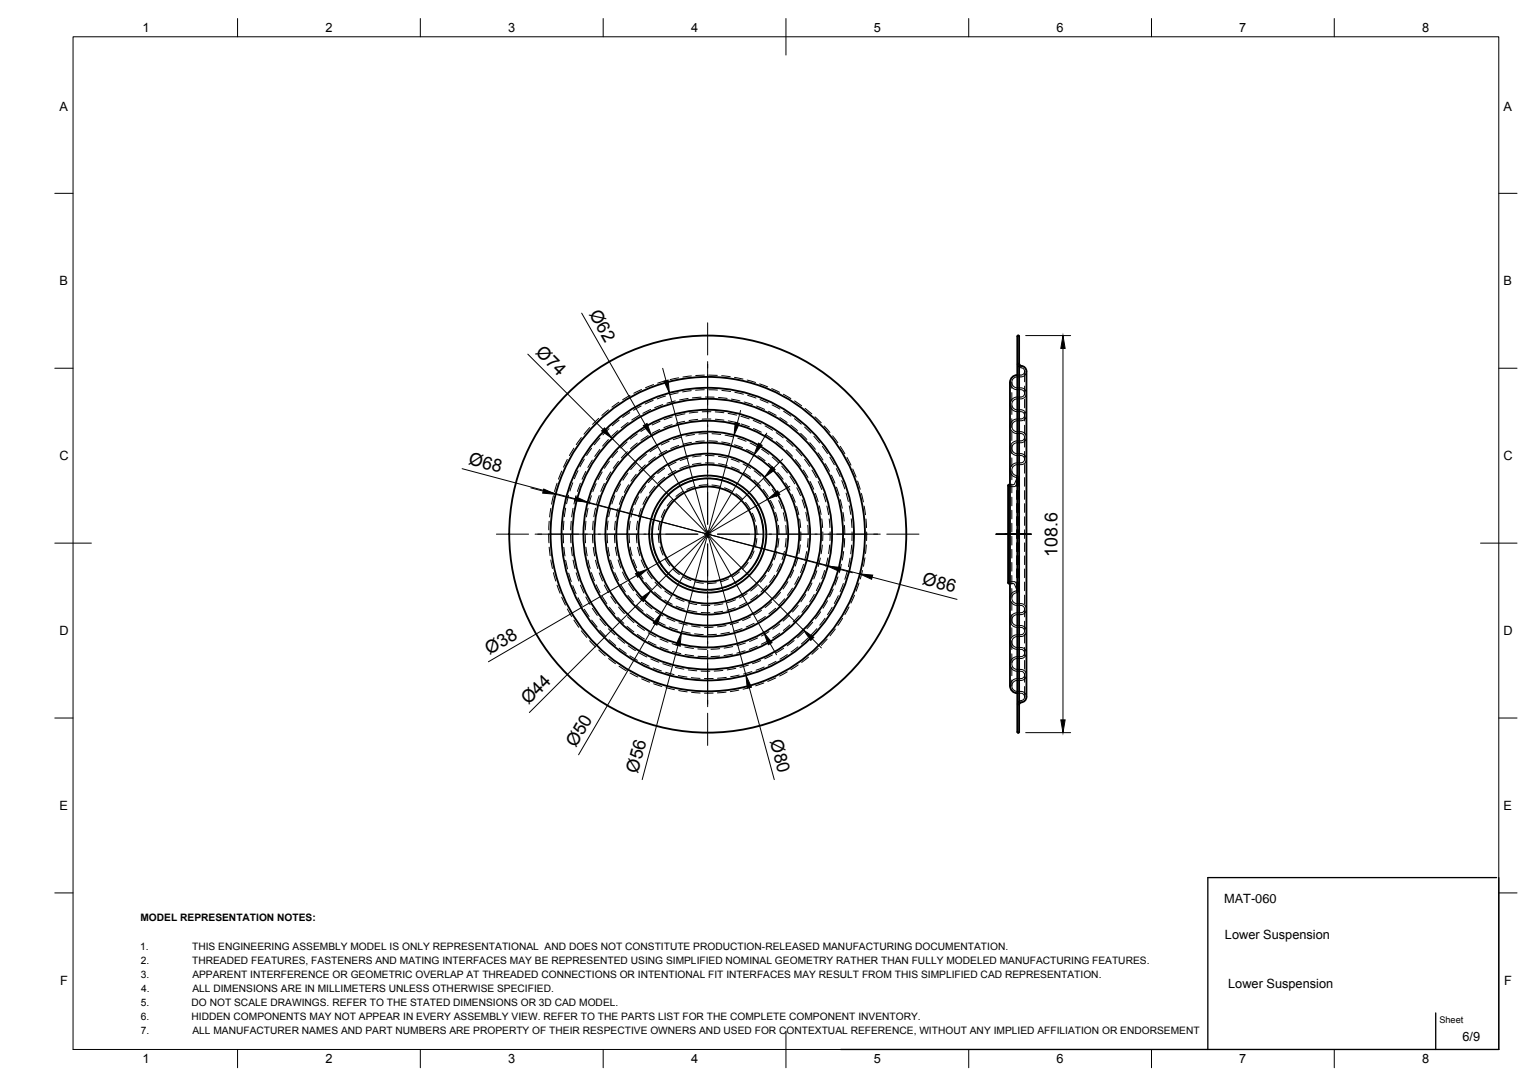
ISO-10303-21;
HEADER;
FILE_DESCRIPTION (('STEP AP214'),
    '1' );
FILE_NAME ('Lower Suspension.step',
    '2026-10-29T23:46:56',
    ( '' ),
    ( '' ),
    'SwSTEP 2.0',
    'SolidWorks 2020',
    '' );
FILE_SCHEMA (( 'AUTOMOTIVE_DESIGN' ));
ENDSEC;

DATA;
#3=CARTESIAN_POINT ( 'NONE',  ( -8.402144023942796025, 14.86454579224779948, 47.04930799450052348 ) ) ;
#7=DIRECTION ( 'NONE',  ( -0.000000000000000000, -1.000000000000000000, 0.000000000000000000 ) ) ;
#16=CIRCLE ( 'NONE', #21997, 37.50000000000000711 ) ;
#18=EDGE_CURVE ( 'NONE', #23289, #31921, #28501, .T. ) ;
#33=EDGE_CURVE ( 'NONE', #28622, #18652, #13708, .T. ) ;
#61=DIRECTION ( 'NONE',  ( -0.000000000000000000, -1.000000000000000000, 0.000000000000000000 ) ) ;
#105=CYLINDRICAL_SURFACE ( 'NONE', #15721, 33.50000000000000000 ) ;
#126=EDGE_CURVE ( 'NONE', #12313, #19851, #23434, .T. ) ;
#127=FACE_OUTER_BOUND ( 'NONE', #2532, .T. ) ;
#144=AXIS2_PLACEMENT_3D ( 'NONE', #10705, #31040, #25937 ) ;
#148=DIRECTION ( 'NONE',  ( -1.000000000000000000, 0.000000000000000000, 0.000000000000000000 ) ) ;
#159=CARTESIAN_POINT ( 'NONE',  ( 21.09785597605720753, 14.86454579224779948, 47.04930799450052348 ) ) ;
#160=CARTESIAN_POINT ( 'NONE',  ( 75.19785597605721250, 14.66454579224780019, 47.04930799450051637 ) ) ;
#161=EDGE_CURVE ( 'NONE', #17230, #26186, #19107, .T. ) ;
#163=VERTEX_POINT ( 'NONE', #26839 ) ;
#164=ORIENTED_EDGE ( 'NONE', *, *, #2840, .T. ) ;
#166=FACE_OUTER_BOUND ( 'NONE', #10063, .T. ) ;
#169=ORIENTED_EDGE ( 'NONE', *, *, #20266, .F. ) ;
#198=CIRCLE ( 'NONE', #29008, 34.00000000000000000 ) ;
#201=EDGE_CURVE ( 'NONE', #31745, #29739, #32095, .T. ) ;
#212=CARTESIAN_POINT ( 'NONE',  ( 21.09785597605720753, 15.23835801850285776, 47.04930799450052348 ) ) ;
#227=FACE_OUTER_BOUND ( 'NONE', #31629, .T. ) ;
#233=DIRECTION ( 'NONE',  ( -1.000000000000000000, 0.000000000000000000, 0.000000000000000000 ) ) ;
#234=AXIS2_PLACEMENT_3D ( 'NONE', #13203, #26134, #3648 ) ;
#238=ORIENTED_EDGE ( 'NONE', *, *, #2347, .F. ) ;
#241=AXIS2_PLACEMENT_3D ( 'NONE', #30077, #17255, #27274 ) ;
#242=AXIS2_PLACEMENT_3D ( 'NONE', #2741, #20287, #4883 ) ;
#243=DIRECTION ( 'NONE',  ( 0.000000000000000000, 0.000000000000000000, 1.000000000000000000 ) ) ;
#247=CARTESIAN_POINT ( 'NONE',  ( 42.59785597605719687, 13.86454579224779948, 47.04930799450052348 ) ) ;
#275=CARTESIAN_POINT ( 'NONE',  ( 64.59785597605720397, 13.86454579224779948, 47.04930799450051637 ) ) ;
#285=DIRECTION ( 'NONE',  ( -0.000000000000000000, -1.000000000000000000, 0.000000000000000000 ) ) ;
#294=VERTEX_POINT ( 'NONE', #26940 ) ;
#297=ORIENTED_EDGE ( 'NONE', *, *, #25455, .T. ) ;
#315=DIRECTION ( 'NONE',  ( -0.000000000000000000, -1.000000000000000000, 0.000000000000000000 ) ) ;
#319=DIRECTION ( 'NONE',  ( -1.224646799147353207E-16, 0.000000000000000000, -1.000000000000000000 ) ) ;
#332=DIRECTION ( 'NONE',  ( -0.000000000000000000, -1.000000000000000000, 0.000000000000000000 ) ) ;
#339=DIRECTION ( 'NONE',  ( -1.000000000000000000, 0.000000000000000000, 0.000000000000000000 ) ) ;
#344=DIRECTION ( 'NONE',  ( -0.000000000000000000, -1.000000000000000000, 0.000000000000000000 ) ) ;
#345=AXIS2_PLACEMENT_3D ( 'NONE', #21627, #16382, #28696 ) ;
#354=SURFACE_STYLE_FILL_AREA ( #4142 ) ;
#364=DIRECTION ( 'NONE',  ( -1.000000000000000000, 0.000000000000000000, 0.000000000000000000 ) ) ;
#374=CARTESIAN_POINT ( 'NONE',  ( -25.43703420551703687, 14.86454579224779948, 47.04930799450052348 ) ) ;
#380=CARTESIAN_POINT ( 'NONE',  ( -33.00214402394279745, 14.56454579224780055, 47.04930799450052348 ) ) ;
#385=DIRECTION ( 'NONE',  ( -0.000000000000000000, -1.000000000000000000, 0.000000000000000000 ) ) ;
#393=DIRECTION ( 'NONE',  ( -0.000000000000000000, -1.000000000000000000, 0.000000000000000000 ) ) ;
#399=ORIENTED_EDGE ( 'NONE', *, *, #19336, .T. ) ;
#402=VECTOR ( 'NONE', #29431, 1000.000000000000000 ) ;
#416=ADVANCED_FACE ( 'NONE', ( #13916 ), #14557, .T. ) ;
#419=CIRCLE ( 'NONE', #21369, 34.00000000000000000 ) ;
#431=ORIENTED_EDGE ( 'NONE', *, *, #27668, .F. ) ;
#455=CIRCLE ( 'NONE', #23507, 1.290569415042103207 ) ;
#463=CIRCLE ( 'NONE', #20375, 0.3999999999999975797 ) ;
#470=EDGE_LOOP ( 'NONE', ( #9443, #11981, #20479, #1663 ) ) ;
#490=VERTEX_POINT ( 'NONE', #19471 ) ;
#492=AXIS2_PLACEMENT_3D ( 'NONE', #30621, #8133, #15667 ) ;
#500=EDGE_LOOP ( 'NONE', ( #31319, #977, #18838, #21612 ) ) ;
#524=FACE_OUTER_BOUND ( 'NONE', #6231, .T. ) ;
#547=AXIS2_PLACEMENT_3D ( 'NONE', #22754, #7337, #22261 ) ;
#548=VECTOR ( 'NONE', #4777, 1000.000000000000000 ) ;
#572=DIRECTION ( 'NONE',  ( -0.000000000000000000, -1.000000000000000000, 0.000000000000000000 ) ) ;
#581=AXIS2_PLACEMENT_3D ( 'NONE', #5824, #5343, #30613 ) ;
#616=ADVANCED_FACE ( 'NONE', ( #14724 ), #105, .F. ) ;
#617=DIRECTION ( 'NONE',  ( -1.000000000000000000, 0.000000000000000000, 0.000000000000000000 ) ) ;
#620=EDGE_LOOP ( 'NONE', ( #3859, #30417, #14895, #17526 ) ) ;
#627=ORIENTED_EDGE ( 'NONE', *, *, #27698, .T. ) ;
#629=TOROIDAL_SURFACE ( 'NONE', #20027, 35.50000000000000711, 2.000000000000001776 ) ;
#634=DIRECTION ( 'NONE',  ( 0.000000000000000000, 0.000000000000000000, 1.000000000000000000 ) ) ;
#646=VECTOR ( 'NONE', #22286, 1000.000000000000000 ) ;
#659=ORIENTED_EDGE ( 'NONE', *, *, #25819, .T. ) ;
#663=VERTEX_POINT ( 'NONE', #19058 ) ;
#665=VERTEX_POINT ( 'NONE', #23832 ) ;
#676=DIRECTION ( 'NONE',  ( -1.000000000000000000, 0.000000000000000000, 0.000000000000000000 ) ) ;
#678=DIRECTION ( 'NONE',  ( -0.000000000000000000, -1.000000000000000000, 0.000000000000000000 ) ) ;
#692=VECTOR ( 'NONE', #11554, 1000.000000000000000 ) ;
#706=CARTESIAN_POINT ( 'NONE',  ( 21.09785597605720753, 14.86454579224779948, 47.04930799450052348 ) ) ;
#710=EDGE_CURVE ( 'NONE', #26545, #16815, #18901, .T. ) ;
#733=CARTESIAN_POINT ( 'NONE',  ( -4.402144023942796025, 14.86454579224779948, 47.04930799450052348 ) ) ;
#742=DIRECTION ( 'NONE',  ( -1.000000000000000000, 0.000000000000000000, 0.000000000000000000 ) ) ;
#745=ORIENTED_EDGE ( 'NONE', *, *, #29770, .T. ) ;
#764=EDGE_LOOP ( 'NONE', ( #11253, #25732, #6784, #15942 ) ) ;
#772=DIRECTION ( 'NONE',  ( -1.224646799147353207E-16, 0.000000000000000000, -1.000000000000000000 ) ) ;
#775=DIRECTION ( 'NONE',  ( -0.000000000000000000, -1.000000000000000000, 0.000000000000000000 ) ) ;
#783=AXIS2_PLACEMENT_3D ( 'NONE', #18069, #31044, #28097 ) ;
#795=TOROIDAL_SURFACE ( 'NONE', #23343, 14.00178401536290806, 0.5000000000000004441 ) ;
#801=AXIS2_PLACEMENT_3D ( 'NONE', #9771, #4184, #12401 ) ;
#817=DIRECTION ( 'NONE',  ( -0.000000000000000000, -1.000000000000000000, 0.000000000000000000 ) ) ;
#826=ORIENTED_EDGE ( 'NONE', *, *, #5317, .F. ) ;
#829=DIRECTION ( 'NONE',  ( -1.224646799147353207E-16, 0.000000000000000000, -1.000000000000000000 ) ) ;
#847=CARTESIAN_POINT ( 'NONE',  ( 61.09785597605719687, 13.86454579224779948, 47.04930799450051637 ) ) ;
#861=EDGE_LOOP ( 'NONE', ( #24263, #7176, #5578, #9165 ) ) ;
#878=CARTESIAN_POINT ( 'NONE',  ( 67.13598395589038148, 13.95840365082257151, 47.04930799450051637 ) ) ;
#890=EDGE_CURVE ( 'NONE', #8606, #20520, #3192, .T. ) ;
#896=ORIENTED_EDGE ( 'NONE', *, *, #11025, .F. ) ;
#904=TOROIDAL_SURFACE ( 'NONE', #1959, 20.49999999999999645, 0.9999999999999974465 ) ;
#927=DIRECTION ( 'NONE',  ( 0.000000000000000000, 0.000000000000000000, 1.000000000000000000 ) ) ;
#953=EDGE_LOOP ( 'NONE', ( #21634, #23029, #10824, #21413 ) ) ;
#956=CIRCLE ( 'NONE', #32436, 40.00000000000000711 ) ;
#977=ORIENTED_EDGE ( 'NONE', *, *, #26692, .T. ) ;
#985=DIRECTION ( 'NONE',  ( -1.000000000000000000, 0.000000000000000000, 0.000000000000000000 ) ) ;
#996=ORIENTED_EDGE ( 'NONE', *, *, #8934, .T. ) ;
#1013=VERTEX_POINT ( 'NONE', #8550 ) ;
#1023=DIRECTION ( 'NONE',  ( -0.000000000000000000, -1.000000000000000000, 0.000000000000000000 ) ) ;
#1025=AXIS2_PLACEMENT_3D ( 'NONE', #1697, #21378, #8608 ) ;
#1049=CARTESIAN_POINT ( 'NONE',  ( 21.09785597605720753, 13.86454579224779948, 47.04930799450052348 ) ) ;
#1051=DIRECTION ( 'NONE',  ( -0.000000000000000000, -1.000000000000000000, 0.000000000000000000 ) ) ;
#1052=ORIENTED_EDGE ( 'NONE', *, *, #17154, .F. ) ;
#1079=CARTESIAN_POINT ( 'NONE',  ( 49.09785597605720397, 13.86454579224779948, 47.04930799450052348 ) ) ;
#1095=AXIS2_PLACEMENT_3D ( 'NONE', #18592, #20746, #15506 ) ;
#1102=ORIENTED_EDGE ( 'NONE', *, *, #890, .T. ) ;
#1120=CIRCLE ( 'NONE', #24168, 15.28675991284684343 ) ;
#1158=VERTEX_POINT ( 'NONE', #19679 ) ;
#1159=DIRECTION ( 'NONE',  ( -0.000000000000000000, -1.000000000000000000, 0.000000000000000000 ) ) ;
#1160=AXIS2_PLACEMENT_3D ( 'NONE', #19272, #11903, #31929 ) ;
#1191=EDGE_LOOP ( 'NONE', ( #20839, #14385, #18300, #16135 ) ) ;
#1192=CARTESIAN_POINT ( 'NONE',  ( 60.59785597605720397, 14.86454579224779948, 47.04930799450051637 ) ) ;
#1196=MANIFOLD_SOLID_BREP ( 'Stock-MAT-060-1', #11089 ) ;
#1206=LINE ( 'NONE', #30777, #8886 ) ;
#1212=ORIENTED_EDGE ( 'NONE', *, *, #28402, .T. ) ;
#1218=CONICAL_SURFACE ( 'NONE', #30581, 13.20165371409683708, 1.570144820418440945 ) ;
#1225=CIRCLE ( 'NONE', #32177, 46.53489018157424084 ) ;
#1227=FACE_OUTER_BOUND ( 'NONE', #10320, .T. ) ;
#1231=CARTESIAN_POINT ( 'NONE',  ( 61.09785597605721108, -5.098646251524523443, 47.04930799450051637 ) ) ;
#1242=ORIENTED_EDGE ( 'NONE', *, *, #28098, .T. ) ;
#1245=EDGE_CURVE ( 'NONE', #18233, #24509, #5247, .T. ) ;
#1256=ORIENTED_EDGE ( 'NONE', *, *, #4300, .T. ) ;
#1275=CIRCLE ( 'NONE', #11247, 46.03812797983318461 ) ;
#1281=CARTESIAN_POINT ( 'NONE',  ( 21.09785597605720753, 14.86454579224779948, 47.04930799450052348 ) ) ;
#1296=EDGE_CURVE ( 'NONE', #19168, #20299, #21078, .T. ) ;
#1321=DIRECTION ( 'NONE',  ( -0.000000000000000000, -1.000000000000000000, 0.000000000000000000 ) ) ;
#1332=AXIS2_PLACEMENT_3D ( 'NONE', #5299, #12197, #17433 ) ;
#1354=DIRECTION ( 'NONE',  ( 0.000000000000000000, 0.000000000000000000, 1.000000000000000000 ) ) ;
#1363=CARTESIAN_POINT ( 'NONE',  ( 21.09785597605720753, 15.11603238453479037, 47.04930799450052348 ) ) ;
#1377=CIRCLE ( 'NONE', #13975, 33.50000000000000000 ) ;
#1380=CIRCLE ( 'NONE', #19729, 54.10000000000000142 ) ;
#1387=DIRECTION ( 'NONE',  ( -1.000000000000000000, 0.000000000000000000, 0.000000000000000000 ) ) ;
#1388=ORIENTED_EDGE ( 'NONE', *, *, #25283, .F. ) ;
#1403=CARTESIAN_POINT ( 'NONE',  ( 59.59785597605720397, 13.86454579224779948, 47.04930799450051637 ) ) ;
#1415=ORIENTED_EDGE ( 'NONE', *, *, #9403, .T. ) ;
#1417=EDGE_LOOP ( 'NONE', ( #27072, #20083, #10401, #7399 ) ) ;
#1419=AXIS2_PLACEMENT_3D ( 'NONE', #21368, #5980, #13693 ) ;
#1426=CYLINDRICAL_SURFACE ( 'NONE', #18100, 34.00000000000000000 ) ;
#1432=ADVANCED_FACE ( 'NONE', ( #21127 ), #14282, .T. ) ;
#1433=ORIENTED_EDGE ( 'NONE', *, *, #18374, .T. ) ;
#1434=CARTESIAN_POINT ( 'NONE',  ( -33.20214402394279318, 14.66454579224779842, 47.04930799450052348 ) ) ;
#1437=CARTESIAN_POINT ( 'NONE',  ( 21.09785597605720753, 14.86454579224779948, 47.04930799450052348 ) ) ;
#1482=DIRECTION ( 'NONE',  ( -1.000000000000000000, 0.000000000000000000, 0.000000000000000000 ) ) ;
#1483=FACE_OUTER_BOUND ( 'NONE', #28820, .T. ) ;
#1488=CARTESIAN_POINT ( 'NONE',  ( 67.79048676704638865, 13.68462854903246573, 47.04930799450051637 ) ) ;
#1505=CARTESIAN_POINT ( 'NONE',  ( 7.596071960694297687, -5.098646251524523443, 47.04930799450052348 ) ) ;
#1514=CYLINDRICAL_SURFACE ( 'NONE', #21014, 54.30000000000000426 ) ;
#1522=CARTESIAN_POINT ( 'NONE',  ( 5.811096063210362317, 14.98269195386757602, 47.04930799450052348 ) ) ;
#1532=ORIENTED_EDGE ( 'NONE', *, *, #7122, .T. ) ;
#1537=ORIENTED_EDGE ( 'NONE', *, *, #16167, .F. ) ;
#1543=CYLINDRICAL_SURFACE ( 'NONE', #29774, 31.50000000000000000 ) ;
#1560=DIRECTION ( 'NONE',  ( -1.000000000000000000, 0.000000000000000000, 0.000000000000000000 ) ) ;
#1566=DIRECTION ( 'NONE',  ( -0.000000000000000000, -1.000000000000000000, 0.000000000000000000 ) ) ;
#1569=TOROIDAL_SURFACE ( 'NONE', #2111, 41.50000000000000000, 1.999999999999998224 ) ;
#1573=AXIS2_PLACEMENT_3D ( 'NONE', #2497, #15138, #12523 ) ;
#1585=AXIS2_PLACEMENT_3D ( 'NONE', #20292, #30323, #1560 ) ;
#1589=CYLINDRICAL_SURFACE ( 'NONE', #7623, 25.50000000000000355 ) ;
#1595=ORIENTED_EDGE ( 'NONE', *, *, #19844, .T. ) ;
#1613=DIRECTION ( 'NONE',  ( -0.000000000000000000, -1.000000000000000000, 0.000000000000000000 ) ) ;
#1616=DIRECTION ( 'NONE',  ( -0.000000000000000000, -1.000000000000000000, 0.000000000000000000 ) ) ;
#1618=ORIENTED_EDGE ( 'NONE', *, *, #5754, .T. ) ;
#1650=CYLINDRICAL_SURFACE ( 'NONE', #30215, 13.50178401536290806 ) ;
#1659=FACE_OUTER_BOUND ( 'NONE', #30379, .T. ) ;
#1663=ORIENTED_EDGE ( 'NONE', *, *, #18980, .T. ) ;
#1664=AXIS2_PLACEMENT_3D ( 'NONE', #2940, #17556, #20664 ) ;
#1692=CARTESIAN_POINT ( 'NONE',  ( 21.09785597605720753, 13.86454579224779948, 47.04930799450052348 ) ) ;
#1697=CARTESIAN_POINT ( 'NONE',  ( 21.09785597605720753, 14.86454579224779948, 47.04930799450052348 ) ) ;
#1705=EDGE_CURVE ( 'NONE', #3673, #7331, #3796, .T. ) ;
#1709=EDGE_CURVE ( 'NONE', #3673, #31872, #30548, .T. ) ;
#1719=CARTESIAN_POINT ( 'NONE',  ( 21.09785597605720753, 14.81645899701909563, 47.04930799450052348 ) ) ;
#1762=ORIENTED_EDGE ( 'NONE', *, *, #31648, .F. ) ;
#1768=DIRECTION ( 'NONE',  ( -0.000000000000000000, -1.000000000000000000, 0.000000000000000000 ) ) ;
#1776=CARTESIAN_POINT ( 'NONE',  ( -4.402144023942796025, 13.86454579224779948, 47.04930799450052348 ) ) ;
#1796=VERTEX_POINT ( 'NONE', #23083 ) ;
#1815=EDGE_CURVE ( 'NONE', #27059, #10602, #6898, .T. ) ;
#1835=ORIENTED_EDGE ( 'NONE', *, *, #9572, .T. ) ;
#1845=AXIS2_PLACEMENT_3D ( 'NONE', #30690, #5572, #3263 ) ;
#1856=ORIENTED_EDGE ( 'NONE', *, *, #8300, .T. ) ;
#1867=DIRECTION ( 'NONE',  ( 0.000000000000000000, 0.000000000000000000, 1.000000000000000000 ) ) ;
#1868=ORIENTED_EDGE ( 'NONE', *, *, #12433, .F. ) ;
#1875=DIRECTION ( 'NONE',  ( -1.224646799147353207E-16, 0.000000000000000000, -1.000000000000000000 ) ) ;
#1891=EDGE_CURVE ( 'NONE', #26545, #19851, #18412, .T. ) ;
#1902=ORIENTED_EDGE ( 'NONE', *, *, #24442, .T. ) ;
#1933=ORIENTED_EDGE ( 'NONE', *, *, #22375, .F. ) ;
#1935=DIRECTION ( 'NONE',  ( 0.9275012328650846793, -0.3738200944756017163, -1.135861416033449914E-16 ) ) ;
#1959=AXIS2_PLACEMENT_3D ( 'NONE', #7931, #27946, #15149 ) ;
#1971=ORIENTED_EDGE ( 'NONE', *, *, #4751, .T. ) ;
#2003=DIRECTION ( 'NONE',  ( -0.000000000000000000, -1.000000000000000000, 0.000000000000000000 ) ) ;
#2009=AXIS2_PLACEMENT_3D ( 'NONE', #9915, #29946, #12718 ) ;
#2010=AXIS2_PLACEMENT_3D ( 'NONE', #11975, #7046, #4265 ) ;
#2012=DIRECTION ( 'NONE',  ( -0.000000000000000000, -1.000000000000000000, 0.000000000000000000 ) ) ;
#2037=AXIS2_PLACEMENT_3D ( 'NONE', #3, #2629, #15747 ) ;
#2045=CARTESIAN_POINT ( 'NONE',  ( 34.09963999142011204, 15.70210863493540288, 47.04930799450052348 ) ) ;
#2053=CARTESIAN_POINT ( 'NONE',  ( 21.09785597605720753, 14.86454579224779948, 47.04930799450052348 ) ) ;
#2055=DIRECTION ( 'NONE',  ( -0.000000000000000000, -1.000000000000000000, 0.000000000000000000 ) ) ;
#2057=DIRECTION ( 'NONE',  ( -1.000000000000000000, 0.000000000000000000, 0.000000000000000000 ) ) ;
#2061=CIRCLE ( 'NONE', #20397, 27.49999999999999645 ) ;
#2071=ADVANCED_FACE ( 'NONE', ( #24704 ), #30126, .T. ) ;
#2079=DIRECTION ( 'NONE',  ( -1.000000000000000000, 0.000000000000000000, 0.000000000000000000 ) ) ;
#2088=DIRECTION ( 'NONE',  ( -1.224646799147353207E-16, 0.000000000000000000, -1.000000000000000000 ) ) ;
#2111=AXIS2_PLACEMENT_3D ( 'NONE', #4236, #18822, #16688 ) ;
#2112=TOROIDAL_SURFACE ( 'NONE', #7373, 13.30178401536290878, 0.2000000000000002609 ) ;
#2129=ORIENTED_EDGE ( 'NONE', *, *, #16040, .F. ) ;
#2142=CARTESIAN_POINT ( 'NONE',  ( 21.09785597605720753, 17.16467605102632632, 47.04930799450052348 ) ) ;
#2144=AXIS2_PLACEMENT_3D ( 'NONE', #28347, #8003, #23255 ) ;
#2159=EDGE_LOOP ( 'NONE', ( #14206, #9203, #31203, #26392 ) ) ;
#2173=DIRECTION ( 'NONE',  ( 0.000000000000000000, 0.000000000000000000, 1.000000000000000000 ) ) ;
#2182=ADVANCED_FACE ( 'NONE', ( #18269 ), #2727, .T. ) ;
#2186=DIRECTION ( 'NONE',  ( -0.000000000000000000, -1.000000000000000000, 0.000000000000000000 ) ) ;
#2193=ADVANCED_FACE ( 'NONE', ( #8276 ), #25512, .F. ) ;
#2199=CIRCLE ( 'NONE', #20531, 1.999999999999998224 ) ;
#2206=DIRECTION ( 'NONE',  ( -0.000000000000000000, -1.000000000000000000, 0.000000000000000000 ) ) ;
#2208=VECTOR ( 'NONE', #12644, 1000.000000000000000 ) ;
#2217=ORIENTED_EDGE ( 'NONE', *, *, #17290, .F. ) ;
#2219=CARTESIAN_POINT ( 'NONE',  ( 21.09785597605720753, -5.098646251524523443, 47.04930799450052348 ) ) ;
#2228=EDGE_CURVE ( 'NONE', #27481, #12804, #5802, .T. ) ;
#2242=CARTESIAN_POINT ( 'NONE',  ( 21.09785597605720753, -5.098646251524523443, 47.04930799450052348 ) ) ;
#2263=AXIS2_PLACEMENT_3D ( 'NONE', #4002, #14021, #19083 ) ;
#2272=CARTESIAN_POINT ( 'NONE',  ( 58.09785597605721108, -5.098646251524523443, 47.04930799450051637 ) ) ;
#2278=VECTOR ( 'NONE', #21411, 1000.000000000000000 ) ;
#2279=AXIS2_PLACEMENT_3D ( 'NONE', #14814, #20364, #10056 ) ;
#2288=LINE ( 'NONE', #30033, #23866 ) ;
#2307=TOROIDAL_SURFACE ( 'NONE', #26411, 15.35463912851480828, 0.6621856154243856984 ) ;
#2309=FACE_OUTER_BOUND ( 'NONE', #10411, .T. ) ;
#2311=EDGE_CURVE ( 'NONE', #7331, #3673, #14263, .T. ) ;
#2312=VERTEX_POINT ( 'NONE', #20333 ) ;
#2316=LINE ( 'NONE', #32192, #548 ) ;
#2328=ORIENTED_EDGE ( 'NONE', *, *, #25601, .T. ) ;
#2345=ADVANCED_FACE ( 'NONE', ( #27573 ), #1218, .F. ) ;
#2347=EDGE_CURVE ( 'NONE', #16477, #663, #28484, .T. ) ;
#2348=AXIS2_PLACEMENT_3D ( 'NONE', #11822, #13796, #19020 ) ;
#2350=EDGE_LOOP ( 'NONE', ( #17700, #31035, #31048, #18559 ) ) ;
#2353=DIRECTION ( 'NONE',  ( -1.000000000000000000, 0.000000000000000000, 0.000000000000000000 ) ) ;
#2357=AXIS2_PLACEMENT_3D ( 'NONE', #14559, #12104, #2413 ) ;
#2390=FACE_OUTER_BOUND ( 'NONE', #24514, .T. ) ;
#2393=DIRECTION ( 'NONE',  ( 1.000000000000000000, 0.000000000000000000, 0.000000000000000000 ) ) ;
#2407=ADVANCED_FACE ( 'NONE', ( #31327 ), #27966, .T. ) ;
#2413=DIRECTION ( 'NONE',  ( -1.000000000000000000, 0.000000000000000000, 0.000000000000000000 ) ) ;
#2439=EDGE_LOOP ( 'NONE', ( #4209, #25565, #3242, #13634 ) ) ;
#2441=VERTEX_POINT ( 'NONE', #13301 ) ;
#2443=AXIS2_PLACEMENT_3D ( 'NONE', #21790, #26722, #9166 ) ;
#2450=AXIS2_PLACEMENT_3D ( 'NONE', #27101, #16920, #14639 ) ;
#2463=DIRECTION ( 'NONE',  ( -0.000000000000000000, -1.000000000000000000, 0.000000000000000000 ) ) ;
#2468=CARTESIAN_POINT ( 'NONE',  ( -23.40214402394279247, 13.86454579224779948, 47.04930799450052348 ) ) ;
#2480=CARTESIAN_POINT ( 'NONE',  ( 21.09785597605720753, 13.86454579224779948, 47.04930799450052348 ) ) ;
#2491=CYLINDRICAL_SURFACE ( 'NONE', #241, 33.50000000000000000 ) ;
#2497=CARTESIAN_POINT ( 'NONE',  ( 21.09785597605720753, -5.098646251524523443, 47.04930799450052348 ) ) ;
#2507=DIRECTION ( 'NONE',  ( -1.000000000000000000, 0.000000000000000000, 0.000000000000000000 ) ) ;
#2522=ADVANCED_FACE ( 'NONE', ( #21296 ), #8834, .F. ) ;
#2532=EDGE_LOOP ( 'NONE', ( #10022, #23605, #1532, #19365 ) ) ;
#2535=VECTOR ( 'NONE', #22077, 999.9999999999998863 ) ;
#2539=DIRECTION ( 'NONE',  ( -0.000000000000000000, -1.000000000000000000, 0.000000000000000000 ) ) ;
#2546=CARTESIAN_POINT ( 'NONE',  ( 7.796071960694296976, 17.16474120167318418, 47.04930799450052348 ) ) ;
#2556=AXIS2_PLACEMENT_3D ( 'NONE', #29728, #17235, #27250 ) ;
#2557=VERTEX_POINT ( 'NONE', #22112 ) ;
#2560=DIRECTION ( 'NONE',  ( -1.000000000000000000, 0.000000000000000000, 0.000000000000000000 ) ) ;
#2564=ORIENTED_EDGE ( 'NONE', *, *, #1705, .T. ) ;
#2568=DIRECTION ( 'NONE',  ( -1.000000000000000000, 0.000000000000000000, 0.000000000000000000 ) ) ;
#2594=ORIENTED_EDGE ( 'NONE', *, *, #13948, .T. ) ;
#2601=AXIS2_PLACEMENT_3D ( 'NONE', #8776, #28810, #26832 ) ;
#2604=CARTESIAN_POINT ( 'NONE',  ( 53.59785597605720397, 13.86454579224779948, 47.04930799450051637 ) ) ;
#2605=EDGE_CURVE ( 'NONE', #30851, #31921, #18503, .T. ) ;
#2608=DIRECTION ( 'NONE',  ( -0.000000000000000000, -1.000000000000000000, 0.000000000000000000 ) ) ;
#2618=DIRECTION ( 'NONE',  ( -1.000000000000000000, 0.000000000000000000, 0.000000000000000000 ) ) ;
#2621=DIRECTION ( 'NONE',  ( -1.000000000000000000, 0.000000000000000000, 0.000000000000000000 ) ) ;
#2622=CARTESIAN_POINT ( 'NONE',  ( 21.09785597605720753, 17.36467600858027183, 47.04930799450052348 ) ) ;
#2625=ORIENTED_EDGE ( 'NONE', *, *, #12738, .F. ) ;
#2629=DIRECTION ( 'NONE',  ( 0.000000000000000000, 0.000000000000000000, 1.000000000000000000 ) ) ;
#2644=AXIS2_PLACEMENT_3D ( 'NONE', #17608, #7936, #28271 ) ;
#2652=CARTESIAN_POINT ( 'NONE',  ( 21.09785597605720753, 14.66454579224780019, 47.04930799450052348 ) ) ;
#2655=CIRCLE ( 'NONE', #5803, 0.7000000000000061728 ) ;
#2657=CARTESIAN_POINT ( 'NONE',  ( -10.40214402394279425, 13.86454579224779948, 47.04930799450052348 ) ) ;
#2673=ORIENTED_EDGE ( 'NONE', *, *, #22568, .T. ) ;
#2676=CARTESIAN_POINT ( 'NONE',  ( 49.09785597605721108, 14.86454579224779948, 47.04930799450052348 ) ) ;
#2677=ORIENTED_EDGE ( 'NONE', *, *, #17420, .F. ) ;
#2684=FACE_OUTER_BOUND ( 'NONE', #6076, .T. ) ;
#2690=TOROIDAL_SURFACE ( 'NONE', #18398, 15.35463912851480828, 0.6621856154243856984 ) ;
#2691=ORIENTED_EDGE ( 'NONE', *, *, #8934, .F. ) ;
#2702=ORIENTED_EDGE ( 'NONE', *, *, #9200, .T. ) ;
#2727=TOROIDAL_SURFACE ( 'NONE', #20011, 46.53489018157424084, 0.7000000000000002887 ) ;
#2741=CARTESIAN_POINT ( 'NONE',  ( 21.09785597605720753, 14.86454579224779948, 47.04930799450052348 ) ) ;
#2742=DIRECTION ( 'NONE',  ( 1.000000000000000000, 0.000000000000000000, 0.000000000000000000 ) ) ;
#2749=CARTESIAN_POINT ( 'NONE',  ( 61.09785597605721108, 14.86454579224779948, 47.04930799450051637 ) ) ;
#2752=DIRECTION ( 'NONE',  ( -0.000000000000000000, -1.000000000000000000, 0.000000000000000000 ) ) ;
#2759=EDGE_LOOP ( 'NONE', ( #15121, #5548, #3395, #3205 ) ) ;
#2765=AXIS2_PLACEMENT_3D ( 'NONE', #6248, #21011, #30882 ) ;
#2780=EDGE_CURVE ( 'NONE', #9753, #22946, #5965, .T. ) ;
#2782=DIRECTION ( 'NONE',  ( -1.000000000000000000, 0.000000000000000000, 0.000000000000000000 ) ) ;
#2787=SHAPE_DEFINITION_REPRESENTATION ( #24763, #11371 ) ;
#2824=DIRECTION ( 'NONE',  ( -0.000000000000000000, -1.000000000000000000, 0.000000000000000000 ) ) ;
#2827=ORIENTED_EDGE ( 'NONE', *, *, #23066, .F. ) ;
#2834=EDGE_CURVE ( 'NONE', #15810, #12910, #13422, .T. ) ;
#2840=EDGE_CURVE ( 'NONE', #1796, #6385, #12255, .T. ) ;
#2841=CARTESIAN_POINT ( 'NONE',  ( -22.40214402394279247, 14.86454579224779948, 47.04930799450052348 ) ) ;
#2849=ORIENTED_EDGE ( 'NONE', *, *, #4751, .F. ) ;
#2851=DIRECTION ( 'NONE',  ( -1.000000000000000000, 0.000000000000000000, 0.000000000000000000 ) ) ;
#2868=DIRECTION ( 'NONE',  ( -1.224646799147353207E-16, 0.000000000000000000, -1.000000000000000000 ) ) ;
#2870=ORIENTED_EDGE ( 'NONE', *, *, #30114, .F. ) ;
#2876=DIRECTION ( 'NONE',  ( -1.224646799147353207E-16, 0.000000000000000000, -1.000000000000000000 ) ) ;
#2890=EDGE_LOOP ( 'NONE', ( #24943, #20819, #3048, #15004 ) ) ;
#2912=EDGE_LOOP ( 'NONE', ( #31676, #1868, #13955, #3623 ) ) ;
#2929=EDGE_CURVE ( 'NONE', #21091, #11329, #12266, .T. ) ;
#2938=CARTESIAN_POINT ( 'NONE',  ( 21.09785597605720753, 13.78442380691147839, 47.04930799450052348 ) ) ;
#2940=CARTESIAN_POINT ( 'NONE',  ( 21.09785597605720753, 13.80129159329807287, 47.04930799450052348 ) ) ;
#2954=AXIS2_PLACEMENT_3D ( 'NONE', #24614, #4762, #4587 ) ;
#2962=FACE_OUTER_BOUND ( 'NONE', #5982, .T. ) ;
#2985=EDGE_LOOP ( 'NONE', ( #4919, #1388, #31234, #29479 ) ) ;
#2986=ORIENTED_EDGE ( 'NONE', *, *, #710, .T. ) ;
#2992=ADVANCED_FACE ( 'NONE', ( #6504 ), #2307, .T. ) ;
#2993=CIRCLE ( 'NONE', #20277, 2.000000000000001776 ) ;
#3006=DIRECTION ( 'NONE',  ( -1.000000000000000000, 0.000000000000000000, 0.000000000000000000 ) ) ;
#3007=DIRECTION ( 'NONE',  ( -0.000000000000000000, -1.000000000000000000, 0.000000000000000000 ) ) ;
#3013=CIRCLE ( 'NONE', #23981, 22.00000000000000000 ) ;
#3041=EDGE_LOOP ( 'NONE', ( #31383, #31666, #14852, #21465 ) ) ;
#3045=CARTESIAN_POINT ( 'NONE',  ( 21.09785597605720753, 13.95840365082257151, 47.04930799450052348 ) ) ;
#3048=ORIENTED_EDGE ( 'NONE', *, *, #2780, .F. ) ;
#3052=DIRECTION ( 'NONE',  ( -1.000000000000000000, 0.000000000000000000, 0.000000000000000000 ) ) ;
#3060=DIRECTION ( 'NONE',  ( -1.000000000000000000, 0.000000000000000000, 0.000000000000000000 ) ) ;
#3063=AXIS2_PLACEMENT_3D ( 'NONE', #26093, #16082, #6241 ) ;
#3080=CARTESIAN_POINT ( 'NONE',  ( -14.40214402394279780, 14.86454579224779948, 47.04930799450052348 ) ) ;
#3085=ORIENTED_EDGE ( 'NONE', *, *, #30114, .T. ) ;
#3105=DIRECTION ( 'NONE',  ( -0.000000000000000000, -1.000000000000000000, 0.000000000000000000 ) ) ;
#3107=EDGE_CURVE ( 'NONE', #3673, #2441, #17504, .T. ) ;
#3110=EDGE_CURVE ( 'NONE', #13235, #26545, #31136, .T. ) ;
#3114=EDGE_LOOP ( 'NONE', ( #20878, #24219, #4831, #4347 ) ) ;
#3192=CIRCLE ( 'NONE', #7919, 19.00000000000000000 ) ;
#3205=ORIENTED_EDGE ( 'NONE', *, *, #15041, .F. ) ;
#3242=ORIENTED_EDGE ( 'NONE', *, *, #29491, .F. ) ;
#3244=AXIS2_PLACEMENT_3D ( 'NONE', #7279, #17273, #2507 ) ;
#3248=AXIS2_PLACEMENT_3D ( 'NONE', #29635, #4356, #22230 ) ;
#3259=EDGE_CURVE ( 'NONE', #17919, #18936, #20629, .T. ) ;
#3263=DIRECTION ( 'NONE',  ( -1.000000000000000000, 0.000000000000000000, 0.000000000000000000 ) ) ;
#3267=CARTESIAN_POINT ( 'NONE',  ( 21.09785597605720753, 14.16454579224779842, 47.04930799450052348 ) ) ;
#3285=CYLINDRICAL_SURFACE ( 'NONE', #7179, 22.00000000000000000 ) ;
#3296=EDGE_CURVE ( 'NONE', #23946, #25889, #5451, .T. ) ;
#3333=CARTESIAN_POINT ( 'NONE',  ( 75.39785597605721534, 14.56454579224780232, 47.04930799450051637 ) ) ;
#3345=CARTESIAN_POINT ( 'NONE',  ( -15.90214402394279958, 13.86454579224779948, 47.04930799450052348 ) ) ;
#3361=EDGE_CURVE ( 'NONE', #12208, #15228, #6136, .T. ) ;
#3374=DIRECTION ( 'NONE',  ( -0.000000000000000000, -1.000000000000000000, 0.000000000000000000 ) ) ;
#3378=EDGE_LOOP ( 'NONE', ( #399, #10481, #30354, #20357 ) ) ;
#3395=ORIENTED_EDGE ( 'NONE', *, *, #31507, .F. ) ;
#3399=TOROIDAL_SURFACE ( 'NONE', #27514, 15.27594751018003194, 0.2551199516247882326 ) ;
#3403=ADVANCED_FACE ( 'NONE', ( #28954 ), #19237, .T. ) ;
#3423=AXIS2_PLACEMENT_3D ( 'NONE', #16638, #4015, #27148 ) ;
#3431=CARTESIAN_POINT ( 'NONE',  ( -6.902144023942789808, 13.86454579224779948, 47.04930799450052348 ) ) ;
#3432=CARTESIAN_POINT ( 'NONE',  ( 21.09785597605720753, 17.36467600858027183, 47.04930799450052348 ) ) ;
#3443=ADVANCED_FACE ( 'NONE', ( #6298 ), #14015, .T. ) ;
#3489=CARTESIAN_POINT ( 'NONE',  ( -25.43703420551703687, 14.16454579224779842, 47.04930799450052348 ) ) ;
#3518=EDGE_CURVE ( 'NONE', #25493, #16293, #19371, .T. ) ;
#3556=VECTOR ( 'NONE', #1616, 1000.000000000000000 ) ;
#3581=AXIS2_PLACEMENT_3D ( 'NONE', #8277, #28146, #10753 ) ;
#3586=VERTEX_POINT ( 'NONE', #2676 ) ;
#3597=DIRECTION ( 'NONE',  ( -0.000000000000000000, -1.000000000000000000, 0.000000000000000000 ) ) ;
#3609=AXIS2_PLACEMENT_3D ( 'NONE', #10434, #4734, #12129 ) ;
#3618=EDGE_CURVE ( 'NONE', #18804, #31321, #17268, .T. ) ;
#3623=ORIENTED_EDGE ( 'NONE', *, *, #6150, .T. ) ;
#3636=ORIENTED_EDGE ( 'NONE', *, *, #13642, .F. ) ;
#3648=DIRECTION ( 'NONE',  ( -1.000000000000000000, 0.000000000000000000, 0.000000000000000000 ) ) ;
#3673=VERTEX_POINT ( 'NONE', #25483 ) ;
#3688=CARTESIAN_POINT ( 'NONE',  ( 21.09785597605720753, 13.61454579224779771, 47.04930799450052348 ) ) ;
#3716=CARTESIAN_POINT ( 'NONE',  ( 3.597855976057204419, 14.86454579224779948, 47.04930799450052348 ) ) ;
#3753=DIRECTION ( 'NONE',  ( -1.000000000000000000, 0.000000000000000000, 0.000000000000000000 ) ) ;
#3774=CARTESIAN_POINT ( 'NONE',  ( 21.09785597605720753, 15.23758267881771111, 47.04930799450052348 ) ) ;
#3791=DIRECTION ( 'NONE',  ( -1.000000000000000000, 0.000000000000000000, 0.000000000000000000 ) ) ;
#3796=CIRCLE ( 'NONE', #8014, 45.99866570866061011 ) ;
#3815=EDGE_LOOP ( 'NONE', ( #26910, #21990, #8716, #2870 ) ) ;
#3816=LINE ( 'NONE', #12019, #20735 ) ;
#3825=CARTESIAN_POINT ( 'NONE',  ( 46.59785597605721108, 14.86454579224779948, 47.04930799450052348 ) ) ;
#3857=EDGE_LOOP ( 'NONE', ( #5635, #21578, #18371, #28721 ) ) ;
#3859=ORIENTED_EDGE ( 'NONE', *, *, #4413, .F. ) ;
#3869=ORIENTED_EDGE ( 'NONE', *, *, #21978, .F. ) ;
#3880=FACE_OUTER_BOUND ( 'NONE', #26735, .T. ) ;
#3882=EDGE_LOOP ( 'NONE', ( #19031, #25314, #19077, #25480 ) ) ;
#3883=UNCERTAINTY_MEASURE_WITH_UNIT (LENGTH_MEASURE( 1.000000000000000082E-05 ), #21486, 'distance_accuracy_value', 'NONE');
#3892=VERTEX_POINT ( 'NONE', #21841 ) ;
#3904=DIRECTION ( 'NONE',  ( -1.224646799147353207E-16, 0.000000000000000000, -1.000000000000000000 ) ) ;
#3924=CARTESIAN_POINT ( 'NONE',  ( 21.09785597605720753, 13.86454579224779948, 47.04930799450052348 ) ) ;
#3937=CARTESIAN_POINT ( 'NONE',  ( -12.40214402394279603, 14.86454579224779948, 47.04930799450052348 ) ) ;
#3941=CIRCLE ( 'NONE', #18095, 46.27992121592387065 ) ;
#3960=ORIENTED_EDGE ( 'NONE', *, *, #23675, .T. ) ;
#3970=ADVANCED_FACE ( 'NONE', ( #13297 ), #30429, .T. ) ;
#3982=EDGE_CURVE ( 'NONE', #13490, #18781, #6829, .T. ) ;
#3990=CIRCLE ( 'NONE', #24964, 40.00000000000000000 ) ;
#4002=CARTESIAN_POINT ( 'NONE',  ( 21.09785597605720753, 13.86454579224779948, 47.04930799450052348 ) ) ;
#4015=DIRECTION ( 'NONE',  ( -0.000000000000000000, -1.000000000000000000, 0.000000000000000000 ) ) ;
#4025=DIRECTION ( 'NONE',  ( -1.000000000000000000, 0.000000000000000000, 0.000000000000000000 ) ) ;
#4036=EDGE_LOOP ( 'NONE', ( #5706, #21425, #18800, #10206 ) ) ;
#4038=EDGE_CURVE ( 'NONE', #18056, #7765, #31988, .T. ) ;
#4041=ORIENTED_EDGE ( 'NONE', *, *, #9572, .F. ) ;
#4045=CIRCLE ( 'NONE', #1419, 1.999999999999998224 ) ;
#4061=CARTESIAN_POINT ( 'NONE',  ( 21.09785597605720753, -5.098646251524523443, 47.04930799450052348 ) ) ;
#4072=ADVANCED_FACE ( 'NONE', ( #16370 ), #1569, .T. ) ;
#4077=AXIS2_PLACEMENT_3D ( 'NONE', #6217, #16219, #3753 ) ;
#4086=CARTESIAN_POINT ( 'NONE',  ( 52.59785597605720397, -5.098646251524523443, 47.04930799450051637 ) ) ;
#4088=CIRCLE ( 'NONE', #24519, 0.9999999999999940048 ) ;
#4142=FILL_AREA_STYLE ('',( #7099 ) ) ;
#4182=ADVANCED_BREP_SHAPE_REPRESENTATION ( '', ( #1196, #8172 ), #27017 ) ;
#4183=LINE ( 'NONE', #8632, #8426 ) ;
#4184=DIRECTION ( 'NONE',  ( -0.000000000000000000, -1.000000000000000000, 0.000000000000000000 ) ) ;
#4186=DIRECTION ( 'NONE',  ( 0.000000000000000000, 0.000000000000000000, 1.000000000000000000 ) ) ;
#4196=LINE ( 'NONE', #14218, #2278 ) ;
#4207=EDGE_LOOP ( 'NONE', ( #21113, #24059, #31568, #17443 ) ) ;
#4208=AXIS2_PLACEMENT_3D ( 'NONE', #30602, #385, #8112 ) ;
#4209=ORIENTED_EDGE ( 'NONE', *, *, #4708, .T. ) ;
#4236=CARTESIAN_POINT ( 'NONE',  ( 21.09785597605720753, 14.86454579224779948, 47.04930799450052348 ) ) ;
#4246=CARTESIAN_POINT ( 'NONE',  ( 60.59785597605719687, -5.098646251524523443, 47.04930799450051637 ) ) ;
#4253=TOROIDAL_SURFACE ( 'NONE', #27835, 14.00178401536290806, 0.5000000000000004441 ) ;
#4261=DIRECTION ( 'NONE',  ( -0.000000000000000000, -1.000000000000000000, 0.000000000000000000 ) ) ;
#4265=DIRECTION ( 'NONE',  ( -1.000000000000000000, 0.000000000000000000, 0.000000000000000000 ) ) ;
#4300=EDGE_CURVE ( 'NONE', #18077, #2557, #8928, .T. ) ;
#4325=ORIENTED_EDGE ( 'NONE', *, *, #15361, .T. ) ;
#4346=EDGE_CURVE ( 'NONE', #28560, #5653, #22920, .T. ) ;
#4347=ORIENTED_EDGE ( 'NONE', *, *, #33, .F. ) ;
#4354=DIRECTION ( 'NONE',  ( -1.000000000000000000, 0.000000000000000000, 0.000000000000000000 ) ) ;
#4355=DIRECTION ( 'NONE',  ( -1.000000000000000000, 0.000000000000000000, 0.000000000000000000 ) ) ;
#4356=DIRECTION ( 'NONE',  ( -0.000000000000000000, -1.000000000000000000, 0.000000000000000000 ) ) ;
#4360=DIRECTION ( 'NONE',  ( -0.000000000000000000, -1.000000000000000000, 0.000000000000000000 ) ) ;
#4364=ORIENTED_EDGE ( 'NONE', *, *, #17818, .T. ) ;
#4365=LINE ( 'NONE', #4856, #30847 ) ;
#4375=ADVANCED_FACE ( 'NONE', ( #25236 ), #22762, .T. ) ;
#4410=CARTESIAN_POINT ( 'NONE',  ( 65.59785597605720397, 13.86454579224779948, 47.04930799450051637 ) ) ;
#4413=EDGE_CURVE ( 'NONE', #29185, #26331, #2655, .T. ) ;
#4424=MECHANICAL_DESIGN_GEOMETRIC_PRESENTATION_REPRESENTATION('',(#22245),#10615);
#4452=CIRCLE ( 'NONE', #28032, 0.2000000000000005107 ) ;
#4456=CIRCLE ( 'NONE', #16491, 1.500000000000001332 ) ;
#4481=AXIS2_PLACEMENT_3D ( 'NONE', #5961, #10573, #20561 ) ;
#4516=CARTESIAN_POINT ( 'NONE',  ( 21.09785597605720753, 14.86454579224779948, 47.04930799450052348 ) ) ;
#4536=EDGE_CURVE ( 'NONE', #19129, #4851, #18365, .T. ) ;
#4542=DIRECTION ( 'NONE',  ( -0.000000000000000000, -1.000000000000000000, 0.000000000000000000 ) ) ;
#4587=DIRECTION ( 'NONE',  ( -1.000000000000000000, 0.000000000000000000, 0.000000000000000000 ) ) ;
#4613=AXIS2_PLACEMENT_3D ( 'NONE', #5219, #15231, #12451 ) ;
#4619=ADVANCED_FACE ( 'NONE', ( #19935 ), #27004, .F. ) ;
#4621=EDGE_LOOP ( 'NONE', ( #28405, #23388, #16140, #21494 ) ) ;
#4636=CIRCLE ( 'NONE', #2009, 0.6621856154243859205 ) ;
#4637=AXIS2_PLACEMENT_3D ( 'NONE', #31998, #14284, #9517 ) ;
#4653=TOROIDAL_SURFACE ( 'NONE', #8334, 17.50000000000000000, 1.499999999999998668 ) ;
#4669=AXIS2_PLACEMENT_3D ( 'NONE', #30855, #25761, #12820 ) ;
#4677=CARTESIAN_POINT ( 'NONE',  ( 42.59785597605720397, -5.098646251524523443, 47.04930799450052348 ) ) ;
#4679=FACE_OUTER_BOUND ( 'NONE', #13222, .T. ) ;
#4692=ORIENTED_EDGE ( 'NONE', *, *, #25803, .F. ) ;
#4708=EDGE_CURVE ( 'NONE', #2312, #665, #10886, .T. ) ;
#4734=DIRECTION ( 'NONE',  ( -0.000000000000000000, -1.000000000000000000, 0.000000000000000000 ) ) ;
#4741=VECTOR ( 'NONE', #27861, 1000.000000000000000 ) ;
#4746=CIRCLE ( 'NONE', #10525, 1.000000000000000888 ) ;
#4751=EDGE_CURVE ( 'NONE', #23541, #10568, #12996, .T. ) ;
#4757=ORIENTED_EDGE ( 'NONE', *, *, #1245, .F. ) ;
#4762=DIRECTION ( 'NONE',  ( -0.000000000000000000, -1.000000000000000000, 0.000000000000000000 ) ) ;
#4777=DIRECTION ( 'NONE',  ( -0.000000000000000000, -1.000000000000000000, 0.000000000000000000 ) ) ;
#4782=EDGE_CURVE ( 'NONE', #26186, #10938, #18199, .T. ) ;
#4784=VERTEX_POINT ( 'NONE', #25514 ) ;
#4788=ORIENTED_EDGE ( 'NONE', *, *, #16837, .F. ) ;
#4789=CIRCLE ( 'NONE', #31529, 27.49999999999999645 ) ;
#4805=CIRCLE ( 'NONE', #7441, 28.00000000000000000 ) ;
#4831=ORIENTED_EDGE ( 'NONE', *, *, #21249, .T. ) ;
#4833=CARTESIAN_POINT ( 'NONE',  ( 21.09785597605720753, 13.86454579224779948, 47.04930799450052348 ) ) ;
#4846=DIRECTION ( 'NONE',  ( -0.000000000000000000, -1.000000000000000000, 0.000000000000000000 ) ) ;
#4851=VERTEX_POINT ( 'NONE', #21535 ) ;
#4856=CARTESIAN_POINT ( 'NONE',  ( -0.9021440239427926944, -5.098646251524523443, 47.04930799450052348 ) ) ;
#4861=EDGE_LOOP ( 'NONE', ( #13996, #17729, #2702, #12207 ) ) ;
#4877=AXIS2_PLACEMENT_3D ( 'NONE', #15051, #5199, #22587 ) ;
#4883=DIRECTION ( 'NONE',  ( -1.000000000000000000, 0.000000000000000000, 0.000000000000000000 ) ) ;
#4902=FACE_OUTER_BOUND ( 'NONE', #11593, .T. ) ;
#4910=VECTOR ( 'NONE', #6339, 1000.000000000000000 ) ;
#4919=ORIENTED_EDGE ( 'NONE', *, *, #29680, .F. ) ;
#4944=EDGE_CURVE ( 'NONE', #27481, #15810, #4045, .T. ) ;
#4966=PRESENTATION_STYLE_ASSIGNMENT (( #7752 ) ) ;
#4976=ORIENTED_EDGE ( 'NONE', *, *, #20377, .F. ) ;
#4996=EDGE_CURVE ( 'NONE', #15058, #10568, #19570, .T. ) ;
#5000=AXIS2_PLACEMENT_3D ( 'NONE', #6651, #4186, #27155 ) ;
#5005=EDGE_LOOP ( 'NONE', ( #15590, #16305, #5185, #14288 ) ) ;
#5018=CYLINDRICAL_SURFACE ( 'NONE', #27313, 25.00000000000000000 ) ;
#5019=ORIENTED_EDGE ( 'NONE', *, *, #14270, .F. ) ;
#5021=CARTESIAN_POINT ( 'NONE',  ( -23.40214402394279247, 13.86454579224779948, 47.04930799450052348 ) ) ;
#5044=CARTESIAN_POINT ( 'NONE',  ( 21.09785597605720753, 15.19538130838178169, 47.04930799450052348 ) ) ;
#5049=EDGE_CURVE ( 'NONE', #11329, #20520, #29756, .T. ) ;
#5061=ORIENTED_EDGE ( 'NONE', *, *, #17980, .F. ) ;
#5068=AXIS2_PLACEMENT_3D ( 'NONE', #13303, #30695, #15576 ) ;
#5073=AXIS2_PLACEMENT_3D ( 'NONE', #10017, #27569, #2618 ) ;
#5102=CARTESIAN_POINT ( 'NONE',  ( 21.09785597605720753, -5.098646251524523443, 47.04930799450052348 ) ) ;
#5141=CARTESIAN_POINT ( 'NONE',  ( 5.570303151842745493, 15.19538130838178169, 47.04930799450052348 ) ) ;
#5150=ORIENTED_EDGE ( 'NONE', *, *, #20964, .F. ) ;
#5185=ORIENTED_EDGE ( 'NONE', *, *, #2834, .T. ) ;
#5186=CIRCLE ( 'NONE', #31397, 1.500000000000001332 ) ;
#5188=ORIENTED_EDGE ( 'NONE', *, *, #4996, .T. ) ;
#5196=VERTEX_POINT ( 'NONE', #1776 ) ;
#5199=DIRECTION ( 'NONE',  ( -0.000000000000000000, -1.000000000000000000, 0.000000000000000000 ) ) ;
#5200=DIRECTION ( 'NONE',  ( -1.000000000000000000, 0.000000000000000000, 0.000000000000000000 ) ) ;
#5219=CARTESIAN_POINT ( 'NONE',  ( 21.09785597605720753, 14.86454579224779948, 47.04930799450052348 ) ) ;
#5224=AXIS2_PLACEMENT_3D ( 'NONE', #3924, #817, #13946 ) ;
#5225=EDGE_CURVE ( 'NONE', #10602, #27059, #26611, .T. ) ;
#5232=TOROIDAL_SURFACE ( 'NONE', #1025, 41.50000000000000000, 1.999999999999998224 ) ;
#5247=LINE ( 'NONE', #22310, #2208 ) ;
#5252=CARTESIAN_POINT ( 'NONE',  ( 21.09785597605720753, 13.86454579224779948, 47.04930799450052348 ) ) ;
#5258=CARTESIAN_POINT ( 'NONE',  ( 21.09785597605720753, -5.098646251524523443, 47.04930799450052348 ) ) ;
#5267=AXIS2_PLACEMENT_3D ( 'NONE', #6888, #4261, #14281 ) ;
#5274=EDGE_CURVE ( 'NONE', #5196, #17364, #30826, .T. ) ;
#5293=CIRCLE ( 'NONE', #24657, 43.00000000000000000 ) ;
#5299=CARTESIAN_POINT ( 'NONE',  ( 21.09785597605720753, 14.86454579224779948, 47.04930799450052348 ) ) ;
#5300=AXIS2_PLACEMENT_3D ( 'NONE', #13848, #11224, #6460 ) ;
#5304=ORIENTED_EDGE ( 'NONE', *, *, #13286, .T. ) ;
#5317=EDGE_CURVE ( 'NONE', #6385, #8606, #21628, .T. ) ;
#5330=CARTESIAN_POINT ( 'NONE',  ( 67.03037309312014713, 14.61319044934410627, 47.04930799450051637 ) ) ;
#5343=DIRECTION ( 'NONE',  ( -0.000000000000000000, -1.000000000000000000, 0.000000000000000000 ) ) ;
#5392=CIRCLE ( 'NONE', #25295, 22.00000000000000000 ) ;
#5420=ADVANCED_FACE ( 'NONE', ( #7687 ), #7774, .F. ) ;
#5431=CARTESIAN_POINT ( 'NONE',  ( -24.94027200377598064, 13.95840365082257151, 47.04930799450052348 ) ) ;
#5432=AXIS2_PLACEMENT_3D ( 'NONE', #24844, #7772, #29608 ) ;
#5440=EDGE_LOOP ( 'NONE', ( #8085, #2849, #20025, #15254 ) ) ;
#5445=EDGE_CURVE ( 'NONE', #26196, #10005, #17680, .T. ) ;
#5451=CIRCLE ( 'NONE', #30080, 37.00000000000000711 ) ;
#5460=CARTESIAN_POINT ( 'NONE',  ( 58.59785597605721108, 14.86454579224779948, 47.04930799450051637 ) ) ;
#5461=EDGE_CURVE ( 'NONE', #17919, #29185, #455, .T. ) ;
#5479=CYLINDRICAL_SURFACE ( 'NONE', #22820, 39.49999999999999289 ) ;
#5496=EDGE_CURVE ( 'NONE', #10005, #12804, #26126, .T. ) ;
#5510=VERTEX_POINT ( 'NONE', #23421 ) ;
#5511=CARTESIAN_POINT ( 'NONE',  ( 59.59785597605720397, 13.86454579224779948, 47.04930799450051637 ) ) ;
#5519=DIRECTION ( 'NONE',  ( -0.000000000000000000, -1.000000000000000000, 0.000000000000000000 ) ) ;
#5532=ORIENTED_EDGE ( 'NONE', *, *, #13948, .F. ) ;
#5548=ORIENTED_EDGE ( 'NONE', *, *, #2347, .T. ) ;
#5550=TOROIDAL_SURFACE ( 'NONE', #32277, 38.50000000000000000, 1.499999999999997780 ) ;
#5566=EDGE_LOOP ( 'NONE', ( #896, #10859, #27346, #8860 ) ) ;
#5572=DIRECTION ( 'NONE',  ( -0.000000000000000000, -1.000000000000000000, 0.000000000000000000 ) ) ;
#5578=ORIENTED_EDGE ( 'NONE', *, *, #3518, .T. ) ;
#5589=EDGE_CURVE ( 'NONE', #20520, #8606, #10416, .T. ) ;
#5602=CIRCLE ( 'NONE', #25536, 34.00000000000000000 ) ;
#5621=ORIENTED_EDGE ( 'NONE', *, *, #3518, .F. ) ;
#5633=DIRECTION ( 'NONE',  ( -1.000000000000000000, 0.000000000000000000, 0.000000000000000000 ) ) ;
#5635=ORIENTED_EDGE ( 'NONE', *, *, #27109, .F. ) ;
#5645=ORIENTED_EDGE ( 'NONE', *, *, #26692, .F. ) ;
#5651=DIRECTION ( 'NONE',  ( -0.000000000000000000, -1.000000000000000000, 0.000000000000000000 ) ) ;
#5653=VERTEX_POINT ( 'NONE', #16029 ) ;
#5703=AXIS2_PLACEMENT_3D ( 'NONE', #8366, #18363, #15916 ) ;
#5706=ORIENTED_EDGE ( 'NONE', *, *, #22038, .F. ) ;
#5727=ORIENTED_EDGE ( 'NONE', *, *, #27675, .F. ) ;
#5737=DIRECTION ( 'NONE',  ( -0.000000000000000000, -1.000000000000000000, 0.000000000000000000 ) ) ;
#5750=AXIS2_PLACEMENT_3D ( 'NONE', #18917, #26639, #14181 ) ;
#5753=EDGE_CURVE ( 'NONE', #7619, #6508, #4365, .T. ) ;
#5754=EDGE_CURVE ( 'NONE', #10875, #12313, #12083, .T. ) ;
#5760=CIRCLE ( 'NONE', #17816, 16.00569570871410008 ) ;
#5778=ORIENTED_EDGE ( 'NONE', *, *, #33, .T. ) ;
#5786=CIRCLE ( 'NONE', #4208, 19.50000000000000000 ) ;
#5801=CARTESIAN_POINT ( 'NONE',  ( -15.90214402394279958, -5.098646251524523443, 47.04930799450052348 ) ) ;
#5802=CIRCLE ( 'NONE', #28343, 0.2551199516247883436 ) ;
#5803=AXIS2_PLACEMENT_3D ( 'NONE', #26352, #21580, #31451 ) ;
#5824=CARTESIAN_POINT ( 'NONE',  ( 21.09785597605720753, 15.70210863493540288, 47.04930799450052348 ) ) ;
#5844=TOROIDAL_SURFACE ( 'NONE', #6343, 32.50000000000000000, 1.499999999999999556 ) ;
#5853=AXIS2_PLACEMENT_3D ( 'NONE', #26513, #16647, #4025 ) ;
#5872=ORIENTED_EDGE ( 'NONE', *, *, #11025, .T. ) ;
#5898=AXIS2_PLACEMENT_3D ( 'NONE', #30684, #16367, #23122 ) ;
#5899=CARTESIAN_POINT ( 'NONE',  ( 21.09785597605720753, 13.68462854903246573, 47.04930799450052348 ) ) ;
#5902=VECTOR ( 'NONE', #14264, 1000.000000000000000 ) ;
#5914=ORIENTED_EDGE ( 'NONE', *, *, #1709, .F. ) ;
#5923=CARTESIAN_POINT ( 'NONE',  ( 21.09785597605720753, -5.098646251524523443, 47.04930799450052348 ) ) ;
#5940=ORIENTED_EDGE ( 'NONE', *, *, #25803, .T. ) ;
#5961=CARTESIAN_POINT ( 'NONE',  ( 36.37380348623724302, 15.23758267881771111, 47.04930799450052348 ) ) ;
#5965=CIRCLE ( 'NONE', #11729, 37.50000000000000711 ) ;
#5977=DIRECTION ( 'NONE',  ( 1.000000000000000000, 0.000000000000000000, 0.000000000000000000 ) ) ;
#5980=DIRECTION ( 'NONE',  ( 0.000000000000000000, 0.000000000000000000, 1.000000000000000000 ) ) ;
#5982=EDGE_LOOP ( 'NONE', ( #28899, #745, #6137, #18708 ) ) ;
#5983=CARTESIAN_POINT ( 'NONE',  ( 21.09785597605720753, 14.86454579224779948, 47.04930799450052348 ) ) ;
#5985=DIRECTION ( 'NONE',  ( -0.000000000000000000, -1.000000000000000000, 0.000000000000000000 ) ) ;
#5998=CARTESIAN_POINT ( 'NONE',  ( 21.09785597605720753, 14.86454579224779948, 47.04930799450052348 ) ) ;
#6008=AXIS2_PLACEMENT_3D ( 'NONE', #23985, #32198, #19212 ) ;
#6012=CARTESIAN_POINT ( 'NONE',  ( 21.09785597605720753, 14.86454579224779948, 47.04930799450052348 ) ) ;
#6027=ORIENTED_EDGE ( 'NONE', *, *, #6410, .T. ) ;
#6030=CARTESIAN_POINT ( 'NONE',  ( 21.09785597605720753, 13.86454579224779948, 47.04930799450052348 ) ) ;
#6037=CIRCLE ( 'NONE', #242, 43.50000000000000000 ) ;
#6038=CIRCLE ( 'NONE', #7081, 1.500000000000001332 ) ;
#6046=ADVANCED_FACE ( 'NONE', ( #23856 ), #5232, .T. ) ;
#6057=VECTOR ( 'NONE', #25979, 1000.000000000000114 ) ;
#6076=EDGE_LOOP ( 'NONE', ( #16530, #10990, #31310, #11925 ) ) ;
#6082=EDGE_LOOP ( 'NONE', ( #7343, #22582, #11643, #27869 ) ) ;
#6090=CARTESIAN_POINT ( 'NONE',  ( 21.09785597605720753, 14.36454579224779948, 47.04930799450052348 ) ) ;
#6095=AXIS2_PLACEMENT_3D ( 'NONE', #19361, #1321, #24295 ) ;
#6105=CARTESIAN_POINT ( 'NONE',  ( 21.09785597605720753, 14.66454579224779842, 47.04930799450052348 ) ) ;
#6111=DIRECTION ( 'NONE',  ( -0.000000000000000000, -1.000000000000000000, 0.000000000000000000 ) ) ;
#6121=CIRCLE ( 'NONE', #2450, 1.499999999999997780 ) ;
#6124=FACE_OUTER_BOUND ( 'NONE', #470, .T. ) ;
#6125=DIRECTION ( 'NONE',  ( -0.000000000000000000, -1.000000000000000000, 0.000000000000000000 ) ) ;
#6128=FACE_OUTER_BOUND ( 'NONE', #19991, .T. ) ;
#6133=ORIENTED_EDGE ( 'NONE', *, *, #4782, .F. ) ;
#6136=LINE ( 'NONE', #31096, #17490 ) ;
#6137=ORIENTED_EDGE ( 'NONE', *, *, #8490, .T. ) ;
#6144=CARTESIAN_POINT ( 'NONE',  ( 21.09785597605720753, -5.098646251524523443, 47.04930799450052348 ) ) ;
#6150=EDGE_CURVE ( 'NONE', #12910, #163, #18313, .T. ) ;
#6159=ORIENTED_EDGE ( 'NONE', *, *, #29491, .T. ) ;
#6161=CARTESIAN_POINT ( 'NONE',  ( 21.09785597605720753, 14.86454579224779948, 47.04930799450052348 ) ) ;
#6187=ORIENTED_EDGE ( 'NONE', *, *, #890, .F. ) ;
#6190=VECTOR ( 'NONE', #344, 1000.000000000000000 ) ;
#6196=CARTESIAN_POINT ( 'NONE',  ( 21.09785597605720753, 16.03967147762301693, 47.04930799450052348 ) ) ;
#6208=FACE_OUTER_BOUND ( 'NONE', #28664, .T. ) ;
#6212=DIRECTION ( 'NONE',  ( -0.000000000000000000, -1.000000000000000000, 0.000000000000000000 ) ) ;
#6217=CARTESIAN_POINT ( 'NONE',  ( 21.09785597605720753, 13.86454579224779948, 47.04930799450052348 ) ) ;
#6231=EDGE_LOOP ( 'NONE', ( #5621, #1242, #30904, #5150 ) ) ;
#6240=ORIENTED_EDGE ( 'NONE', *, *, #24482, .F. ) ;
#6241=DIRECTION ( 'NONE',  ( -1.000000000000000000, 0.000000000000000000, 0.000000000000000000 ) ) ;
#6248=CARTESIAN_POINT ( 'NONE',  ( 21.09785597605720753, 13.78442380691147839, 47.04930799450052348 ) ) ;
#6254=DIRECTION ( 'NONE',  ( -1.000000000000000000, 0.000000000000000000, 0.000000000000000000 ) ) ;
#6258=CARTESIAN_POINT ( 'NONE',  ( 21.09785597605720753, 14.86454579224779948, 47.04930799450052348 ) ) ;
#6267=DIRECTION ( 'NONE',  ( -0.000000000000000000, -1.000000000000000000, 0.000000000000000000 ) ) ;
#6278=DIRECTION ( 'NONE',  ( -0.000000000000000000, -1.000000000000000000, 0.000000000000000000 ) ) ;
#6286=CARTESIAN_POINT ( 'NONE',  ( 0.000000000000000000, 0.000000000000000000, 0.000000000000000000 ) ) ;
#6294=ORIENTED_EDGE ( 'NONE', *, *, #5049, .T. ) ;
#6296=DIRECTION ( 'NONE',  ( -1.224646799147353207E-16, 0.000000000000000000, -1.000000000000000000 ) ) ;
#6298=FACE_OUTER_BOUND ( 'NONE', #500, .T. ) ;
#6317=DIRECTION ( 'NONE',  ( -1.000000000000000000, 0.000000000000000000, 0.000000000000000000 ) ) ;
#6339=DIRECTION ( 'NONE',  ( -0.000000000000000000, -1.000000000000000000, 0.000000000000000000 ) ) ;
#6343=AXIS2_PLACEMENT_3D ( 'NONE', #15027, #7799, #20258 ) ;
#6350=ADVANCED_FACE ( 'NONE', ( #1659 ), #8327, .F. ) ;
#6360=ORIENTED_EDGE ( 'NONE', *, *, #3107, .F. ) ;
#6366=EDGE_CURVE ( 'NONE', #25938, #31872, #16687, .T. ) ;
#6375=DIRECTION ( 'NONE',  ( -0.000000000000000000, -1.000000000000000000, 0.000000000000000000 ) ) ;
#6380=CARTESIAN_POINT ( 'NONE',  ( 21.09785597605720753, 14.86454579224779948, 47.04930799450052348 ) ) ;
#6383=AXIS2_PLACEMENT_3D ( 'NONE', #2219, #2539, #17633 ) ;
#6385=VERTEX_POINT ( 'NONE', #7728 ) ;
#6386=DIRECTION ( 'NONE',  ( 1.000000000000000000, 0.000000000000000000, 0.000000000000000000 ) ) ;
#6410=EDGE_CURVE ( 'NONE', #29883, #4784, #24548, .T. ) ;
#6417=EDGE_LOOP ( 'NONE', ( #3636, #26328, #26977, #14469 ) ) ;
#6420=DIRECTION ( 'NONE',  ( -1.000000000000000000, 0.000000000000000000, 0.000000000000000000 ) ) ;
#6441=AXIS2_PLACEMENT_3D ( 'NONE', #1437, #6375, #26396 ) ;
#6460=DIRECTION ( 'NONE',  ( -1.000000000000000000, 0.000000000000000000, 0.000000000000000000 ) ) ;
#6492=CARTESIAN_POINT ( 'NONE',  ( 34.39963999142011630, 17.16474120167318418, 47.04930799450052348 ) ) ;
#6501=CARTESIAN_POINT ( 'NONE',  ( 21.09785597605720753, 13.86454579224779948, 47.04930799450052348 ) ) ;
#6504=FACE_OUTER_BOUND ( 'NONE', #11847, .T. ) ;
#6508=VERTEX_POINT ( 'NONE', #15430 ) ;
#6520=EDGE_CURVE ( 'NONE', #19129, #23289, #28748, .T. ) ;
#6524=DIRECTION ( 'NONE',  ( -1.000000000000000000, 0.000000000000000000, 0.000000000000000000 ) ) ;
#6536=DIRECTION ( 'NONE',  ( -1.000000000000000000, 0.000000000000000000, 0.000000000000000000 ) ) ;
#6556=EDGE_LOOP ( 'NONE', ( #12790, #10963, #28604, #25017 ) ) ;
#6558=AXIS2_PLACEMENT_3D ( 'NONE', #22788, #13443, #15562 ) ;
#6561=DIRECTION ( 'NONE',  ( -1.000000000000000000, 0.000000000000000000, 0.000000000000000000 ) ) ;
#6570=DIRECTION ( 'NONE',  ( -0.000000000000000000, -1.000000000000000000, 0.000000000000000000 ) ) ;
#6582=DIRECTION ( 'NONE',  ( -0.000000000000000000, -1.000000000000000000, 0.000000000000000000 ) ) ;
#6585=ORIENTED_EDGE ( 'NONE', *, *, #12778, .T. ) ;
#6588=ORIENTED_EDGE ( 'NONE', *, *, #20291, .T. ) ;
#6620=DIRECTION ( 'NONE',  ( -1.000000000000000000, 0.000000000000000000, 0.000000000000000000 ) ) ;
#6622=DIRECTION ( 'NONE',  ( -0.000000000000000000, -1.000000000000000000, 0.000000000000000000 ) ) ;
#6630=ADVANCED_FACE ( 'NONE', ( #15752 ), #19833, .F. ) ;
#6643=DIRECTION ( 'NONE',  ( -1.000000000000000000, 0.000000000000000000, 0.000000000000000000 ) ) ;
#6648=CARTESIAN_POINT ( 'NONE',  ( 21.09785597605720753, 14.86454579224779948, 47.04930799450052348 ) ) ;
#6651=CARTESIAN_POINT ( 'NONE',  ( -25.59477481493196294, 13.68462854903246573, 47.04930799450052348 ) ) ;
#6656=DIRECTION ( 'NONE',  ( -1.000000000000000000, 0.000000000000000000, 0.000000000000000000 ) ) ;
#6662=DIRECTION ( 'NONE',  ( -1.224646799147353207E-16, 0.000000000000000000, -1.000000000000000000 ) ) ;
#6670=EDGE_LOOP ( 'NONE', ( #19412, #23972, #29221, #1971 ) ) ;
#6682=DIRECTION ( 'NONE',  ( -0.000000000000000000, -1.000000000000000000, 0.000000000000000000 ) ) ;
#6719=CARTESIAN_POINT ( 'NONE',  ( 46.59785597605721108, -5.098646251524523443, 47.04930799450052348 ) ) ;
#6737=CARTESIAN_POINT ( 'NONE',  ( 21.09785597605720753, -5.098646251524523443, 47.04930799450052348 ) ) ;
#6750=ADVANCED_FACE ( 'NONE', ( #21801 ), #14273, .T. ) ;
#6764=CIRCLE ( 'NONE', #13577, 1.499999999999994449 ) ;
#6765=DIRECTION ( 'NONE',  ( -0.000000000000000000, -1.000000000000000000, 0.000000000000000000 ) ) ;
#6781=AXIS2_PLACEMENT_3D ( 'NONE', #20189, #7727, #17723 ) ;
#6784=ORIENTED_EDGE ( 'NONE', *, *, #1891, .F. ) ;
#6818=EDGE_CURVE ( 'NONE', #7331, #25938, #463, .T. ) ;
#6829=CIRCLE ( 'NONE', #12607, 27.99999999999999645 ) ;
#6848=CARTESIAN_POINT ( 'NONE',  ( 64.59785597605720397, 14.86454579224779948, 47.04930799450051637 ) ) ;
#6859=EDGE_CURVE ( 'NONE', #26186, #23946, #6764, .T. ) ;
#6861=CARTESIAN_POINT ( 'NONE',  ( 21.09785597605720753, 14.86454579224779948, 47.04930799450052348 ) ) ;
#6876=ORIENTED_EDGE ( 'NONE', *, *, #10546, .F. ) ;
#6888=CARTESIAN_POINT ( 'NONE',  ( 21.09785597605720753, 14.86454579224779948, 47.04930799450052348 ) ) ;
#6898=CIRCLE ( 'NONE', #14778, 39.49999999999999289 ) ;
#6906=DIRECTION ( 'NONE',  ( -1.000000000000000000, 0.000000000000000000, 0.000000000000000000 ) ) ;
#6911=DIRECTION ( 'NONE',  ( -1.000000000000000000, 0.000000000000000000, 0.000000000000000000 ) ) ;
#6970=DIRECTION ( 'NONE',  ( -0.000000000000000000, -1.000000000000000000, 0.000000000000000000 ) ) ;
#6972=DIRECTION ( 'NONE',  ( -0.000000000000000000, -1.000000000000000000, 0.000000000000000000 ) ) ;
#6980=DIRECTION ( 'NONE',  ( -0.000000000000000000, -1.000000000000000000, 0.000000000000000000 ) ) ;
#7000=CIRCLE ( 'NONE', #17478, 43.00000000000000000 ) ;
#7033=ADVANCED_FACE ( 'NONE', ( #11391 ), #11240, .T. ) ;
#7037=ORIENTED_EDGE ( 'NONE', *, *, #6859, .T. ) ;
#7046=DIRECTION ( 'NONE',  ( -0.000000000000000000, -1.000000000000000000, 0.000000000000000000 ) ) ;
#7077=AXIS2_PLACEMENT_3D ( 'NONE', #6090, #678, #28254 ) ;
#7081=AXIS2_PLACEMENT_3D ( 'NONE', #2604, #9670, #12633 ) ;
#7097=DIRECTION ( 'NONE',  ( -0.000000000000000000, -1.000000000000000000, 0.000000000000000000 ) ) ;
#7099=FILL_AREA_STYLE_COLOUR ( '', #29650 ) ;
#7100=VERTEX_POINT ( 'NONE', #30106 ) ;
#7117=CARTESIAN_POINT ( 'NONE',  ( 21.09785597605720753, 13.86454579224779948, 47.04930799450052348 ) ) ;
#7122=EDGE_CURVE ( 'NONE', #17663, #16815, #28264, .T. ) ;
#7133=AXIS2_PLACEMENT_3D ( 'NONE', #15327, #2206, #17125 ) ;
#7149=CARTESIAN_POINT ( 'NONE',  ( 21.09785597605720753, 15.11603238453479037, 47.04930799450052348 ) ) ;
#7151=CARTESIAN_POINT ( 'NONE',  ( 34.29950969015404638, 17.36467600858027183, 47.04930799450052348 ) ) ;
#7154=VERTEX_POINT ( 'NONE', #374 ) ;
#7174=DIRECTION ( 'NONE',  ( -0.000000000000000000, -1.000000000000000000, 0.000000000000000000 ) ) ;
#7176=ORIENTED_EDGE ( 'NONE', *, *, #14270, .T. ) ;
#7179=AXIS2_PLACEMENT_3D ( 'NONE', #30869, #22665, #339 ) ;
#7196=ORIENTED_EDGE ( 'NONE', *, *, #2311, .F. ) ;
#7198=AXIS2_PLACEMENT_3D ( 'NONE', #13851, #30932, #20905 ) ;
#7219=FACE_OUTER_BOUND ( 'NONE', #12930, .T. ) ;
#7242=ADVANCED_FACE ( 'NONE', ( #7219 ), #12942, .F. ) ;
#7253=ORIENTED_EDGE ( 'NONE', *, *, #24639, .T. ) ;
#7275=EDGE_CURVE ( 'NONE', #3586, #8390, #17650, .T. ) ;
#7276=CARTESIAN_POINT ( 'NONE',  ( 1.597855976057205973, 13.86454579224779948, 47.04930799450052348 ) ) ;
#7279=CARTESIAN_POINT ( 'NONE',  ( 21.09785597605720753, 14.46497581658974063, 47.04930799450052348 ) ) ;
#7294=CIRCLE ( 'NONE', #2037, 1.500000000000001332 ) ;
#7313=EDGE_LOOP ( 'NONE', ( #21819, #2673, #27185, #18228 ) ) ;
#7331=VERTEX_POINT ( 'NONE', #12314 ) ;
#7335=CARTESIAN_POINT ( 'NONE',  ( 8.096071960694297687, -5.098646251524523443, 47.04930799450052348 ) ) ;
#7337=DIRECTION ( 'NONE',  ( 0.000000000000000000, 0.000000000000000000, 1.000000000000000000 ) ) ;
#7340=ORIENTED_EDGE ( 'NONE', *, *, #5753, .F. ) ;
#7343=ORIENTED_EDGE ( 'NONE', *, *, #22973, .F. ) ;
#7356=EDGE_CURVE ( 'NONE', #10177, #2557, #1380, .T. ) ;
#7373=AXIS2_PLACEMENT_3D ( 'NONE', #27062, #5519, #2560 ) ;
#7399=ORIENTED_EDGE ( 'NONE', *, *, #24984, .T. ) ;
#7410=CIRCLE ( 'NONE', #10032, 15.52755282421446026 ) ;
#7416=ORIENTED_EDGE ( 'NONE', *, *, #18980, .F. ) ;
#7432=FACE_OUTER_BOUND ( 'NONE', #5440, .T. ) ;
#7438=ORIENTED_EDGE ( 'NONE', *, *, #11275, .T. ) ;
#7441=AXIS2_PLACEMENT_3D ( 'NONE', #6861, #27530, #11941 ) ;
#7457=EDGE_CURVE ( 'NONE', #6508, #8606, #6121, .T. ) ;
#7472=DIRECTION ( 'NONE',  ( -0.000000000000000000, -1.000000000000000000, 0.000000000000000000 ) ) ;
#7501=EDGE_LOOP ( 'NONE', ( #20597, #12957, #21382, #5061 ) ) ;
#7510=CARTESIAN_POINT ( 'NONE',  ( 21.09785597605720753, 14.86454579224779948, 47.04930799450052348 ) ) ;
#7525=CYLINDRICAL_SURFACE ( 'NONE', #16085, 37.00000000000000711 ) ;
#7535=ADVANCED_FACE ( 'NONE', ( #25771 ), #3285, .T. ) ;
#7542=ADVANCED_FACE ( 'NONE', ( #8379 ), #15556, .T. ) ;
#7546=FACE_OUTER_BOUND ( 'NONE', #13275, .T. ) ;
#7547=DIRECTION ( 'NONE',  ( -0.000000000000000000, -1.000000000000000000, 0.000000000000000000 ) ) ;
#7601=AXIS2_PLACEMENT_3D ( 'NONE', #24283, #19348, #19836 ) ;
#7619=VERTEX_POINT ( 'NONE', #20684 ) ;
#7623=AXIS2_PLACEMENT_3D ( 'NONE', #8815, #21122, #24073 ) ;
#7667=FACE_OUTER_BOUND ( 'NONE', #31896, .T. ) ;
#7671=DIRECTION ( 'NONE',  ( -0.000000000000000000, -1.000000000000000000, 0.000000000000000000 ) ) ;
#7687=FACE_OUTER_BOUND ( 'NONE', #2985, .T. ) ;
#7690=TOROIDAL_SURFACE ( 'NONE', #7133, 46.75000000000000000, 0.7905694150421007649 ) ;
#7697=ORIENTED_EDGE ( 'NONE', *, *, #24913, .F. ) ;
#7714=PRODUCT_CONTEXT ( 'NONE', #8664, 'mechanical' ) ;
#7722=DIRECTION ( 'NONE',  ( -0.000000000000000000, -1.000000000000000000, 0.000000000000000000 ) ) ;
#7727=DIRECTION ( 'NONE',  ( -0.000000000000000000, -1.000000000000000000, 0.000000000000000000 ) ) ;
#7728=CARTESIAN_POINT ( 'NONE',  ( 2.097855976057206195, 14.86454579224779948, 47.04930799450052348 ) ) ;
#7740=VECTOR ( 'NONE', #2012, 1000.000000000000000 ) ;
#7750=DIRECTION ( 'NONE',  ( 0.000000000000000000, 0.000000000000000000, 1.000000000000000000 ) ) ;
#7752=SURFACE_STYLE_USAGE ( .BOTH. , #10219 ) ;
#7763=CARTESIAN_POINT ( 'NONE',  ( -4.402144023942796025, -5.098646251524523443, 47.04930799450052348 ) ) ;
#7765=VERTEX_POINT ( 'NONE', #3937 ) ;
#7766=ORIENTED_EDGE ( 'NONE', *, *, #13580, .T. ) ;
#7767=CARTESIAN_POINT ( 'NONE',  ( -10.40214402394279425, -5.098646251524523443, 47.04930799450052348 ) ) ;
#7768=EDGE_CURVE ( 'NONE', #19572, #1158, #26576, .T. ) ;
#7772=DIRECTION ( 'NONE',  ( -0.000000000000000000, -1.000000000000000000, 0.000000000000000000 ) ) ;
#7774=TOROIDAL_SURFACE ( 'NONE', #4613, 29.50000000000000355, 1.500000000000001332 ) ;
#7791=DIRECTION ( 'NONE',  ( -1.000000000000000000, 0.000000000000000000, 0.000000000000000000 ) ) ;
#7797=DIRECTION ( 'NONE',  ( -0.000000000000000000, -1.000000000000000000, 0.000000000000000000 ) ) ;
#7799=DIRECTION ( 'NONE',  ( -0.000000000000000000, -1.000000000000000000, 0.000000000000000000 ) ) ;
#7817=CIRCLE ( 'NONE', #4669, 2.000000000000001776 ) ;
#7819=CARTESIAN_POINT ( 'NONE',  ( 36.33160203359362583, 14.46497581658974063, 47.04930799450052348 ) ) ;
#7852=CIRCLE ( 'NONE', #26171, 1.000000000000000888 ) ;
#7863=AXIS2_PLACEMENT_3D ( 'NONE', #14505, #9084, #24498 ) ;
#7864=AXIS2_PLACEMENT_3D ( 'NONE', #21001, #31674, #8858 ) ;
#7865=ORIENTED_EDGE ( 'NONE', *, *, #7768, .F. ) ;
#7868=AXIS2_PLACEMENT_3D ( 'NONE', #21355, #26308, #11214 ) ;
#7899=CIRCLE ( 'NONE', #20998, 21.49999999999999645 ) ;
#7918=AXIS2_PLACEMENT_3D ( 'NONE', #22275, #32305, #9815 ) ;
#7919=AXIS2_PLACEMENT_3D ( 'NONE', #18067, #30076, #676 ) ;
#7931=CARTESIAN_POINT ( 'NONE',  ( 21.09785597605720753, 13.86454579224779948, 47.04930799450052348 ) ) ;
#7936=DIRECTION ( 'NONE',  ( -0.000000000000000000, -1.000000000000000000, 0.000000000000000000 ) ) ;
#7944=AXIS2_PLACEMENT_3D ( 'NONE', #15650, #3007, #7791 ) ;
#7952=ADVANCED_FACE ( 'NONE', ( #25852 ), #32311, .T. ) ;
#7972=DIRECTION ( 'NONE',  ( 1.000000000000000000, 0.000000000000000000, 0.000000000000000000 ) ) ;
#7983=ORIENTED_EDGE ( 'NONE', *, *, #15361, .F. ) ;
#7989=ADVANCED_FACE ( 'NONE', ( #28486 ), #13450, .F. ) ;
#7997=DIRECTION ( 'NONE',  ( -1.000000000000000000, 0.000000000000000000, 0.000000000000000000 ) ) ;
#8003=DIRECTION ( 'NONE',  ( -1.224646799147353207E-16, 0.000000000000000000, -1.000000000000000000 ) ) ;
#8007=CARTESIAN_POINT ( 'NONE',  ( 34.39950969015404780, 17.36474115922713324, 47.04930799450052348 ) ) ;
#8008=DIRECTION ( 'NONE',  ( -1.000000000000000000, 0.000000000000000000, 0.000000000000000000 ) ) ;
#8011=AXIS2_PLACEMENT_3D ( 'NONE', #23643, #28571, #16084 ) ;
#8014=AXIS2_PLACEMENT_3D ( 'NONE', #10302, #30163, #12603 ) ;
#8054=TOROIDAL_SURFACE ( 'NONE', #11182, 32.50000000000000000, 1.000000000000000888 ) ;
#8079=AXIS2_PLACEMENT_3D ( 'NONE', #29640, #24052, #11909 ) ;
#8085=ORIENTED_EDGE ( 'NONE', *, *, #16987, .F. ) ;
#8101=CIRCLE ( 'NONE', #22301, 0.6999999999999992895 ) ;
#8102=AXIS2_PLACEMENT_3D ( 'NONE', #2480, #30066, #25133 ) ;
#8105=DIRECTION ( 'NONE',  ( -1.000000000000000000, 0.000000000000000000, 0.000000000000000000 ) ) ;
#8112=DIRECTION ( 'NONE',  ( -1.000000000000000000, 0.000000000000000000, 0.000000000000000000 ) ) ;
#8123=DIRECTION ( 'NONE',  ( -1.000000000000000000, 0.000000000000000000, 0.000000000000000000 ) ) ;
#8133=DIRECTION ( 'NONE',  ( -0.000000000000000000, -1.000000000000000000, 0.000000000000000000 ) ) ;
#8150=CARTESIAN_POINT ( 'NONE',  ( 37.10355168477130405, 14.99513937955032716, 47.04930799450052348 ) ) ;
#8163=CARTESIAN_POINT ( 'NONE',  ( -12.90214402394279603, -5.098646251524523443, 47.04930799450052348 ) ) ;
#8165=DIRECTION ( 'NONE',  ( -1.000000000000000000, 0.000000000000000000, 0.000000000000000000 ) ) ;
#8166=AXIS2_PLACEMENT_3D ( 'NONE', #23755, #26052, #16361 ) ;
#8172=AXIS2_PLACEMENT_3D ( 'NONE', #6286, #1354, #5977 ) ;
#8174=DIRECTION ( 'NONE',  ( -0.000000000000000000, -1.000000000000000000, 0.000000000000000000 ) ) ;
#8186=CARTESIAN_POINT ( 'NONE',  ( 21.09785597605720753, 14.86454579224779948, 47.04930799450052348 ) ) ;
#8203=CARTESIAN_POINT ( 'NONE',  ( 67.37777719198106752, 14.81645899701909563, 47.04930799450051637 ) ) ;
#8206=DIRECTION ( 'NONE',  ( -0.000000000000000000, -1.000000000000000000, 0.000000000000000000 ) ) ;
#8208=FACE_OUTER_BOUND ( 'NONE', #17964, .T. ) ;
#8214=CIRCLE ( 'NONE', #12413, 1.000000000000000888 ) ;
#8217=ORIENTED_EDGE ( 'NONE', *, *, #13239, .T. ) ;
#8221=CARTESIAN_POINT ( 'NONE',  ( -25.65214402394279247, 13.61454579224779771, 47.04930799450052348 ) ) ;
#8232=ADVANCED_FACE ( 'NONE', ( #227 ), #7690, .F. ) ;
#8247=FACE_OUTER_BOUND ( 'NONE', #26863, .T. ) ;
#8249=ORIENTED_EDGE ( 'NONE', *, *, #7457, .F. ) ;
#8252=EDGE_CURVE ( 'NONE', #26196, #17663, #23908, .T. ) ;
#8258=EDGE_CURVE ( 'NONE', #10938, #26186, #3990, .T. ) ;
#8260=CARTESIAN_POINT ( 'NONE',  ( 21.09785597605720753, -5.098646251524523443, 47.04930799450052348 ) ) ;
#8276=FACE_OUTER_BOUND ( 'NONE', #29547, .T. ) ;
#8277=CARTESIAN_POINT ( 'NONE',  ( 21.09785597605720753, 14.56454579224780232, 47.04930799450052348 ) ) ;
#8291=DIRECTION ( 'NONE',  ( -1.224646799147353207E-16, 0.000000000000000000, -1.000000000000000000 ) ) ;
#8298=DIRECTION ( 'NONE',  ( -0.000000000000000000, -1.000000000000000000, 0.000000000000000000 ) ) ;
#8300=EDGE_CURVE ( 'NONE', #19861, #10177, #11763, .T. ) ;
#8302=CIRCLE ( 'NONE', #25595, 0.1999999999999987899 ) ;
#8319=CARTESIAN_POINT ( 'NONE',  ( 21.09785597605720753, 15.70210863493540288, 47.04930799450052348 ) ) ;
#8327=CONICAL_SURFACE ( 'NONE', #11971, 13.20165371409683708, 1.570144820418440945 ) ;
#8334=AXIS2_PLACEMENT_3D ( 'NONE', #21020, #18875, #13813 ) ;
#8341=DIRECTION ( 'NONE',  ( 1.000000000000000000, 0.000000000000000000, 0.000000000000000000 ) ) ;
#8366=CARTESIAN_POINT ( 'NONE',  ( 21.09785597605720753, 13.86454579224779948, 47.04930799450052348 ) ) ;
#8370=ADVANCED_FACE ( 'NONE', ( #8425 ), #31677, .T. ) ;
#8379=FACE_OUTER_BOUND ( 'NONE', #9291, .T. ) ;
#8389=VECTOR ( 'NONE', #6278, 1000.000000000000000 ) ;
#8390=VERTEX_POINT ( 'NONE', #13514 ) ;
#8410=AXIS2_PLACEMENT_3D ( 'NONE', #1403, #13892, #11586 ) ;
#8425=FACE_OUTER_BOUND ( 'NONE', #2759, .T. ) ;
#8426=VECTOR ( 'NONE', #14368, 1000.000000000000000 ) ;
#8434=DIRECTION ( 'NONE',  ( -0.9275012328650849014, -0.3738200944756011057, 0.000000000000000000 ) ) ;
#8440=DIRECTION ( 'NONE',  ( -0.000000000000000000, -1.000000000000000000, 0.000000000000000000 ) ) ;
#8465=CARTESIAN_POINT ( 'NONE',  ( 41.59785597605720397, 13.86454579224779948, 47.04930799450052348 ) ) ;
#8480=DIRECTION ( 'NONE',  ( -0.000000000000000000, -1.000000000000000000, 0.000000000000000000 ) ) ;
#8490=EDGE_CURVE ( 'NONE', #12822, #19635, #19072, .T. ) ;
#8505=CIRCLE ( 'NONE', #18958, 33.50000000000000000 ) ;
#8506=ORIENTED_EDGE ( 'NONE', *, *, #28574, .F. ) ;
#8511=PRODUCT_DEFINITION ( 'UNKNOWN', '', #29164, #32435 ) ;
#8519=CARTESIAN_POINT ( 'NONE',  ( -25.65214402394279247, 13.61454579224779771, 47.04930799450052348 ) ) ;
#8531=DIRECTION ( 'NONE',  ( -1.224646799147353207E-16, 0.000000000000000000, -1.000000000000000000 ) ) ;
#8550=CARTESIAN_POINT ( 'NONE',  ( 46.09785597605720397, 13.86454579224779948, 47.04930799450052348 ) ) ;
#8555=AXIS2_PLACEMENT_3D ( 'NONE', #8519, #15739, #18512 ) ;
#8576=AXIS2_PLACEMENT_3D ( 'NONE', #14904, #19643, #14571 ) ;
#8606=VERTEX_POINT ( 'NONE', #12182 ) ;
#8608=DIRECTION ( 'NONE',  ( -1.000000000000000000, 0.000000000000000000, 0.000000000000000000 ) ) ;
#8632=CARTESIAN_POINT ( 'NONE',  ( -18.90214402394280313, -5.098646251524523443, 47.04930799450052348 ) ) ;
#8653=ORIENTED_EDGE ( 'NONE', *, *, #11275, .F. ) ;
#8664=APPLICATION_CONTEXT ( 'automotive_design' ) ;
#8667=CIRCLE ( 'NONE', #20709, 13.50178401536290806 ) ;
#8673=ORIENTED_EDGE ( 'NONE', *, *, #201, .F. ) ;
#8674=ORIENTED_EDGE ( 'NONE', *, *, #5445, .F. ) ;
#8699=ORIENTED_EDGE ( 'NONE', *, *, #29493, .F. ) ;
#8700=DIRECTION ( 'NONE',  ( 0.000000000000000000, 0.000000000000000000, 1.000000000000000000 ) ) ;
#8707=ORIENTED_EDGE ( 'NONE', *, *, #9342, .F. ) ;
#8716=ORIENTED_EDGE ( 'NONE', *, *, #5274, .F. ) ;
#8742=DIRECTION ( 'NONE',  ( -1.000000000000000000, 0.000000000000000000, 0.000000000000000000 ) ) ;
#8752=CARTESIAN_POINT ( 'NONE',  ( 21.09785597605720753, 14.86454579224779948, 47.04930799450052348 ) ) ;
#8776=CARTESIAN_POINT ( 'NONE',  ( 21.09785597605720753, -5.098646251524523443, 47.04930799450052348 ) ) ;
#8780=ADVANCED_FACE ( 'NONE', ( #2962 ), #32226, .T. ) ;
#8781=ORIENTED_EDGE ( 'NONE', *, *, #28030, .F. ) ;
#8782=CARTESIAN_POINT ( 'NONE',  ( 34.41272994418231690, 15.23835801850285776, 47.04930799450052348 ) ) ;
#8803=EDGE_CURVE ( 'NONE', #13599, #22237, #4452, .T. ) ;
#8815=CARTESIAN_POINT ( 'NONE',  ( 21.09785597605720753, -5.098646251524523443, 47.04930799450052348 ) ) ;
#8833=DIRECTION ( 'NONE',  ( -0.000000000000000000, -1.000000000000000000, 0.000000000000000000 ) ) ;
#8834=CYLINDRICAL_SURFACE ( 'NONE', #29536, 31.00000000000000000 ) ;
#8836=DIRECTION ( 'NONE',  ( -1.000000000000000000, 0.000000000000000000, 0.000000000000000000 ) ) ;
#8858=DIRECTION ( 'NONE',  ( 1.000000000000000000, 0.000000000000000000, 0.000000000000000000 ) ) ;
#8860=ORIENTED_EDGE ( 'NONE', *, *, #2780, .T. ) ;
#8886=VECTOR ( 'NONE', #25997, 1000.000000000000000 ) ;
#8904=AXIS2_PLACEMENT_3D ( 'NONE', #13006, #7750, #23168 ) ;
#8923=LINE ( 'NONE', #14511, #692 ) ;
#8924=ORIENTED_EDGE ( 'NONE', *, *, #16040, .T. ) ;
#8928=CIRCLE ( 'NONE', #2144, 0.2000000000000057288 ) ;
#8930=ADVANCED_FACE ( 'NONE', ( #26264 ), #23312, .F. ) ;
#8934=EDGE_CURVE ( 'NONE', #19861, #18077, #9159, .T. ) ;
#8953=ORIENTED_EDGE ( 'NONE', *, *, #31910, .F. ) ;
#8961=CARTESIAN_POINT ( 'NONE',  ( -5.402144023942789808, 13.86454579224779948, 47.04930799450052348 ) ) ;
#8967=EDGE_CURVE ( 'NONE', #3586, #18781, #11176, .T. ) ;
#8983=DIRECTION ( 'NONE',  ( -1.000000000000000000, 0.000000000000000000, 0.000000000000000000 ) ) ;
#9005=EDGE_CURVE ( 'NONE', #6385, #11329, #21723, .T. ) ;
#9013=DIRECTION ( 'NONE',  ( -1.000000000000000000, 0.000000000000000000, 0.000000000000000000 ) ) ;
#9015=ORIENTED_EDGE ( 'NONE', *, *, #3618, .T. ) ;
#9025=AXIS2_PLACEMENT_3D ( 'NONE', #24095, #1613, #24261 ) ;
#9051=AXIS2_PLACEMENT_3D ( 'NONE', #17667, #27687, #2742 ) ;
#9068=CARTESIAN_POINT ( 'NONE',  ( -24.99296521467773147, 14.05098971466613023, 47.04930799450052348 ) ) ;
#9080=FACE_OUTER_BOUND ( 'NONE', #3114, .T. ) ;
#9084=DIRECTION ( 'NONE',  ( -0.000000000000000000, -1.000000000000000000, 0.000000000000000000 ) ) ;
#9094=VECTOR ( 'NONE', #27276, 1000.000000000000000 ) ;
#9095=APPLICATION_CONTEXT ( 'automotive_design' ) ;
#9097=AXIS2_PLACEMENT_3D ( 'NONE', #24175, #26482, #26963 ) ;
#9122=EDGE_CURVE ( 'NONE', #294, #9753, #2288, .T. ) ;
#9133=ORIENTED_EDGE ( 'NONE', *, *, #18080, .T. ) ;
#9144=CARTESIAN_POINT ( 'NONE',  ( 1.597855976057205973, 14.86454579224779948, 47.04930799450052348 ) ) ;
#9152=CARTESIAN_POINT ( 'NONE',  ( 8.096071960694297687, 15.70210863493540288, 47.04930799450052348 ) ) ;
#9154=DIRECTION ( 'NONE',  ( -0.000000000000000000, -1.000000000000000000, 0.000000000000000000 ) ) ;
#9159=CIRCLE ( 'NONE', #2348, 54.30000000000000426 ) ;
#9165=ORIENTED_EDGE ( 'NONE', *, *, #21785, .F. ) ;
#9166=DIRECTION ( 'NONE',  ( 1.000000000000000000, 0.000000000000000000, 0.000000000000000000 ) ) ;
#9170=VECTOR ( 'NONE', #332, 1000.000000000000000 ) ;
#9175=CARTESIAN_POINT ( 'NONE',  ( -12.40214402394279603, -5.098646251524523443, 47.04930799450052348 ) ) ;
#9178=CARTESIAN_POINT ( 'NONE',  ( 21.09785597605720753, -5.098646251524523443, 47.04930799450052348 ) ) ;
#9200=EDGE_CURVE ( 'NONE', #10938, #25889, #17569, .T. ) ;
#9203=ORIENTED_EDGE ( 'NONE', *, *, #24975, .F. ) ;
#9207=CIRCLE ( 'NONE', #8166, 43.50000000000000000 ) ;
#9229=DIRECTION ( 'NONE',  ( 0.000000000000000000, 0.000000000000000000, 1.000000000000000000 ) ) ;
#9234=DIRECTION ( 'NONE',  ( 1.000000000000000000, 0.000000000000000000, 0.000000000000000000 ) ) ;
#9246=LINE ( 'NONE', #9408, #19213 ) ;
#9259=AXIS2_PLACEMENT_3D ( 'NONE', #6380, #26886, #8836 ) ;
#9277=DIRECTION ( 'NONE',  ( -0.000000000000000000, -1.000000000000000000, 0.000000000000000000 ) ) ;
#9291=EDGE_LOOP ( 'NONE', ( #24511, #16194, #27320, #25913 ) ) ;
#9297=ADVANCED_FACE ( 'NONE', ( #25576 ), #1589, .T. ) ;
#9342=EDGE_CURVE ( 'NONE', #16815, #12159, #8667, .T. ) ;
#9348=AXIS2_PLACEMENT_3D ( 'NONE', #17404, #15583, #22482 ) ;
#9399=FACE_OUTER_BOUND ( 'NONE', #31772, .T. ) ;
#9403=EDGE_CURVE ( 'NONE', #31921, #30851, #9207, .T. ) ;
#9408=CARTESIAN_POINT ( 'NONE',  ( -33.20214402394279318, -5.098646251524523443, 47.04930799450052348 ) ) ;
#9417=ADVANCED_FACE ( 'NONE', ( #23915 ), #1426, .T. ) ;
#9437=CARTESIAN_POINT ( 'NONE',  ( 21.09785597605720753, -5.098646251524523443, 47.04930799450052348 ) ) ;
#9443=ORIENTED_EDGE ( 'NONE', *, *, #14720, .F. ) ;
#9444=CARTESIAN_POINT ( 'NONE',  ( 43.09785597605720397, 14.86454579224779948, 47.04930799450052348 ) ) ;
#9461=AXIS2_PLACEMENT_3D ( 'NONE', #17555, #27572, #12651 ) ;
#9464=TOROIDAL_SURFACE ( 'NONE', #12092, 23.50000000000000000, 2.000000000000001776 ) ;
#9468=DIRECTION ( 'NONE',  ( -0.000000000000000000, -1.000000000000000000, 0.000000000000000000 ) ) ;
#9504=FACE_OUTER_BOUND ( 'NONE', #21593, .T. ) ;
#9506=CIRCLE ( 'NONE', #32019, 1.000000000000000888 ) ;
#9517=DIRECTION ( 'NONE',  ( -1.000000000000000000, 0.000000000000000000, 0.000000000000000000 ) ) ;
#9533=FACE_OUTER_BOUND ( 'NONE', #26133, .T. ) ;
#9536=ADVANCED_FACE ( 'NONE', ( #14727 ), #32234, .T. ) ;
#9543=EDGE_CURVE ( 'NONE', #13599, #24672, #11773, .T. ) ;
#9566=CARTESIAN_POINT ( 'NONE',  ( 21.09785597605720753, 14.56454579224780055, 47.04930799450052348 ) ) ;
#9572=EDGE_CURVE ( 'NONE', #1013, #11782, #14391, .T. ) ;
#9576=AXIS2_PLACEMENT_3D ( 'NONE', #27704, #10315, #25248 ) ;
#9578=CYLINDRICAL_SURFACE ( 'NONE', #16324, 37.00000000000000711 ) ;
#9580=ORIENTED_EDGE ( 'NONE', *, *, #3107, .T. ) ;
#9612=ORIENTED_EDGE ( 'NONE', *, *, #31875, .F. ) ;
#9613=CARTESIAN_POINT ( 'NONE',  ( 62.59785597605721819, 14.86454579224779948, 47.04930799450051637 ) ) ;
#9622=CIRCLE ( 'NONE', #32158, 15.52755282421446026 ) ;
#9626=EDGE_CURVE ( 'NONE', #31872, #25938, #1275, .T. ) ;
#9642=ORIENTED_EDGE ( 'NONE', *, *, #22038, .T. ) ;
#9666=ORIENTED_EDGE ( 'NONE', *, *, #24639, .F. ) ;
#9670=DIRECTION ( 'NONE',  ( -1.224646799147353207E-16, 0.000000000000000000, -1.000000000000000000 ) ) ;
#9681=VERTEX_POINT ( 'NONE', #20125 ) ;
#9694=ORIENTED_EDGE ( 'NONE', *, *, #11434, .F. ) ;
#9696=DIRECTION ( 'NONE',  ( 0.000000000000000000, 0.000000000000000000, 1.000000000000000000 ) ) ;
#9727=CARTESIAN_POINT ( 'NONE',  ( 21.09785597605720753, 14.05098971466613023, 47.04930799450052348 ) ) ;
#9753=VERTEX_POINT ( 'NONE', #19393 ) ;
#9762=DIRECTION ( 'NONE',  ( -0.000000000000000000, -1.000000000000000000, 0.000000000000000000 ) ) ;
#9771=CARTESIAN_POINT ( 'NONE',  ( 21.09785597605720753, 13.86454579224779948, 47.04930799450052348 ) ) ;
#9800=DIRECTION ( 'NONE',  ( -0.000000000000000000, -1.000000000000000000, 0.000000000000000000 ) ) ;
#9804=DIRECTION ( 'NONE',  ( -0.000000000000000000, -1.000000000000000000, 0.000000000000000000 ) ) ;
#9812=CARTESIAN_POINT ( 'NONE',  ( 21.09785597605720753, 14.86454579224779948, 47.04930799450052348 ) ) ;
#9813=FACE_OUTER_BOUND ( 'NONE', #25403, .T. ) ;
#9815=DIRECTION ( 'NONE',  ( -1.000000000000000000, 0.000000000000000000, 0.000000000000000000 ) ) ;
#9823=CARTESIAN_POINT ( 'NONE',  ( 8.096071960694297687, 17.16467605102632632, 47.04930799450052348 ) ) ;
#9827=ADVANCED_FACE ( 'NONE', ( #1227 ), #19079, .T. ) ;
#9855=CARTESIAN_POINT ( 'NONE',  ( 21.09785597605720753, 14.86454579224779948, 47.04930799450052348 ) ) ;
#9883=FACE_OUTER_BOUND ( 'NONE', #6670, .T. ) ;
#9889=EDGE_LOOP ( 'NONE', ( #8699, #10280, #627, #25078 ) ) ;
#9891=CARTESIAN_POINT ( 'NONE',  ( 21.09785597605720753, 13.86454579224779948, 47.04930799450052348 ) ) ;
#9906=DIRECTION ( 'NONE',  ( -0.000000000000000000, -1.000000000000000000, 0.000000000000000000 ) ) ;
#9915=CARTESIAN_POINT ( 'NONE',  ( 5.743216847542398362, 15.11603238453479037, 47.04930799450052348 ) ) ;
#9919=DIRECTION ( 'NONE',  ( -0.000000000000000000, -1.000000000000000000, 0.000000000000000000 ) ) ;
#9933=CARTESIAN_POINT ( 'NONE',  ( 21.09785597605720753, 14.86454579224779948, 47.04930799450052348 ) ) ;
#9937=DIRECTION ( 'NONE',  ( -1.224646799147353207E-16, 0.000000000000000000, -1.000000000000000000 ) ) ;
#9938=ORIENTED_EDGE ( 'NONE', *, *, #18040, .F. ) ;
#9965=VERTEX_POINT ( 'NONE', #2657 ) ;
#9984=CARTESIAN_POINT ( 'NONE',  ( 21.09785597605720753, -5.098646251524523443, 47.04930799450052348 ) ) ;
#9989=ORIENTED_EDGE ( 'NONE', *, *, #28441, .F. ) ;
#9996=AXIS2_PLACEMENT_3D ( 'NONE', #20899, #23041, #10422 ) ;
#10005=VERTEX_POINT ( 'NONE', #30881 ) ;
#10015=EDGE_CURVE ( 'NONE', #9681, #18953, #12336, .T. ) ;
#10017=CARTESIAN_POINT ( 'NONE',  ( 21.09785597605720753, 14.86454579224779948, 47.04930799450052348 ) ) ;
#10021=CARTESIAN_POINT ( 'NONE',  ( 5.821908465877174699, 15.23758267881771111, 47.04930799450052348 ) ) ;
#10022=ORIENTED_EDGE ( 'NONE', *, *, #23825, .F. ) ;
#10024=DIRECTION ( 'NONE',  ( -0.000000000000000000, -1.000000000000000000, 0.000000000000000000 ) ) ;
#10032=AXIS2_PLACEMENT_3D ( 'NONE', #5044, #15052, #5200 ) ;
#10048=CIRCLE ( 'NONE', #18925, 0.9999999999999956701 ) ;
#10056=DIRECTION ( 'NONE',  ( -1.000000000000000000, 0.000000000000000000, 0.000000000000000000 ) ) ;
#10063=EDGE_LOOP ( 'NONE', ( #23895, #16327, #25537, #1102 ) ) ;
#10131=DIRECTION ( 'NONE',  ( 1.000000000000000000, 0.000000000000000000, 0.000000000000000000 ) ) ;
#10134=ORIENTED_EDGE ( 'NONE', *, *, #10015, .F. ) ;
#10141=CARTESIAN_POINT ( 'NONE',  ( -33.00214402394279745, 14.86454579224779948, 47.04930799450052348 ) ) ;
#10142=DIRECTION ( 'NONE',  ( -0.000000000000000000, -1.000000000000000000, 0.000000000000000000 ) ) ;
#10144=TOROIDAL_SURFACE ( 'NONE', #2263, 32.50000000000000000, 1.000000000000000888 ) ;
#10152=CARTESIAN_POINT ( 'NONE',  ( 21.09785597605720753, 14.86454579224779948, 47.04930799450052348 ) ) ;
#10155=DIRECTION ( 'NONE',  ( -0.000000000000000000, -1.000000000000000000, 0.000000000000000000 ) ) ;
#10177=VERTEX_POINT ( 'NONE', #31204 ) ;
#10206=ORIENTED_EDGE ( 'NONE', *, *, #22890, .F. ) ;
#10215=DIRECTION ( 'NONE',  ( -1.000000000000000000, 0.000000000000000000, 0.000000000000000000 ) ) ;
#10216=CARTESIAN_POINT ( 'NONE',  ( 21.09785597605720753, 14.36454579224779948, 47.04930799450052348 ) ) ;
#10219=SURFACE_SIDE_STYLE ('',( #354 ) ) ;
#10226=AXIS2_PLACEMENT_3D ( 'NONE', #3774, #14118, #29049 ) ;
#10273=DIRECTION ( 'NONE',  ( 0.000000000000000000, 0.000000000000000000, 1.000000000000000000 ) ) ;
#10280=ORIENTED_EDGE ( 'NONE', *, *, #30512, .F. ) ;
#10292=ORIENTED_EDGE ( 'NONE', *, *, #17290, .T. ) ;
#10302=CARTESIAN_POINT ( 'NONE',  ( 21.09785597605720753, 13.80129159329807287, 47.04930799450052348 ) ) ;
#10315=DIRECTION ( 'NONE',  ( -0.000000000000000000, -1.000000000000000000, 0.000000000000000000 ) ) ;
#10320=EDGE_LOOP ( 'NONE', ( #3960, #12972, #9694, #27169 ) ) ;
#10366=CARTESIAN_POINT ( 'NONE',  ( 7.896071960694297509, 17.16467605102632632, 47.04930799450052348 ) ) ;
#10367=LINE ( 'NONE', #27926, #6190 ) ;
#10376=( NAMED_UNIT ( * ) PLANE_ANGLE_UNIT ( ) SI_UNIT ( $, .RADIAN. ) );
#10377=EDGE_LOOP ( 'NONE', ( #4757, #20206, #15068, #22264 ) ) ;
#10392=CIRCLE ( 'NONE', #17701, 0.6999999999999992895 ) ;
#10401=ORIENTED_EDGE ( 'NONE', *, *, #2228, .T. ) ;
#10403=VERTEX_POINT ( 'NONE', #32338 ) ;
#10408=CIRCLE ( 'NONE', #3063, 31.00000000000000000 ) ;
#10411=EDGE_LOOP ( 'NONE', ( #14693, #29571 ) ) ;
#10414=CARTESIAN_POINT ( 'NONE',  ( 21.09785597605720753, 15.23835801850285776, 47.04930799450052348 ) ) ;
#10416=CIRCLE ( 'NONE', #21391, 19.00000000000000000 ) ;
#10422=DIRECTION ( 'NONE',  ( -1.000000000000000000, 0.000000000000000000, 0.000000000000000000 ) ) ;
#10424=DIRECTION ( 'NONE',  ( -0.000000000000000000, -1.000000000000000000, 0.000000000000000000 ) ) ;
#10434=CARTESIAN_POINT ( 'NONE',  ( 21.09785597605720753, 13.86454579224779948, 47.04930799450052348 ) ) ;
#10449=ADVANCED_FACE ( 'NONE', ( #28061 ), #24918, .T. ) ;
#10462=ADVANCED_FACE ( 'NONE', ( #13298 ), #795, .F. ) ;
#10481=ORIENTED_EDGE ( 'NONE', *, *, #18, .T. ) ;
#10485=AXIS2_PLACEMENT_3D ( 'NONE', #28139, #15335, #3006 ) ;
#10513=DIRECTION ( 'NONE',  ( -1.000000000000000000, 0.000000000000000000, 0.000000000000000000 ) ) ;
#10514=CARTESIAN_POINT ( 'NONE',  ( 58.09785597605721108, 14.86454579224779948, 47.04930799450051637 ) ) ;
#10515=DIRECTION ( 'NONE',  ( -1.000000000000000000, 0.000000000000000000, 0.000000000000000000 ) ) ;
#10521=CARTESIAN_POINT ( 'NONE',  ( 46.09785597605720397, -5.098646251524523443, 47.04930799450052348 ) ) ;
#10525=AXIS2_PLACEMENT_3D ( 'NONE', #14306, #24139, #11841 ) ;
#10537=ADVANCED_FACE ( 'NONE', ( #6208 ), #31653, .F. ) ;
#10546=EDGE_CURVE ( 'NONE', #18781, #1013, #12883, .T. ) ;
#10568=VERTEX_POINT ( 'NONE', #29180 ) ;
#10573=DIRECTION ( 'NONE',  ( -1.224646799147353207E-16, 0.000000000000000000, -1.000000000000000000 ) ) ;
#10575=ORIENTED_EDGE ( 'NONE', *, *, #8258, .F. ) ;
#10576=DIRECTION ( 'NONE',  ( 1.000000000000000000, 0.000000000000000000, 0.000000000000000000 ) ) ;
#10597=ORIENTED_EDGE ( 'NONE', *, *, #11602, .T. ) ;
#10599=DIRECTION ( 'NONE',  ( -1.000000000000000000, 0.000000000000000000, 0.000000000000000000 ) ) ;
#10602=VERTEX_POINT ( 'NONE', #26553 ) ;
#10605=FACE_OUTER_BOUND ( 'NONE', #26138, .T. ) ;
#10614=EDGE_CURVE ( 'NONE', #17055, #31760, #13123, .T. ) ;
#10615=( GEOMETRIC_REPRESENTATION_CONTEXT ( 3 ) GLOBAL_UNCERTAINTY_ASSIGNED_CONTEXT ( ( #3883 ) ) GLOBAL_UNIT_ASSIGNED_CONTEXT ( ( #21486, #31840, #24445 ) ) REPRESENTATION_CONTEXT ( 'NONE', 'WORKASPACE' ) );
#10620=VERTEX_POINT ( 'NONE', #10141 ) ;
#10646=LINE ( 'NONE', #15711, #31082 ) ;
#10650=ORIENTED_EDGE ( 'NONE', *, *, #19336, .F. ) ;
#10705=CARTESIAN_POINT ( 'NONE',  ( 21.09785597605720753, 13.86454579224779948, 47.04930799450052348 ) ) ;
#10741=LINE ( 'NONE', #11213, #6057 ) ;
#10748=EDGE_LOOP ( 'NONE', ( #14450, #28468, #18628, #27259 ) ) ;
#10753=DIRECTION ( 'NONE',  ( -1.000000000000000000, 0.000000000000000000, 0.000000000000000000 ) ) ;
#10787=ORIENTED_EDGE ( 'NONE', *, *, #29768, .F. ) ;
#10796=DIRECTION ( 'NONE',  ( -0.000000000000000000, -1.000000000000000000, 0.000000000000000000 ) ) ;
#10811=UNCERTAINTY_MEASURE_WITH_UNIT (LENGTH_MEASURE( 1.000000000000000082E-05 ), #14172, 'distance_accuracy_value', 'NONE');
#10824=ORIENTED_EDGE ( 'NONE', *, *, #3296, .T. ) ;
#10830=CARTESIAN_POINT ( 'NONE',  ( 21.09785597605720753, 16.03967147762300982, 47.04930799450052348 ) ) ;
#10853=FACE_BOUND ( 'NONE', #19610, .T. ) ;
#10859=ORIENTED_EDGE ( 'NONE', *, *, #5225, .F. ) ;
#10875=VERTEX_POINT ( 'NONE', #10947 ) ;
#10884=TOROIDAL_SURFACE ( 'NONE', #11398, 35.50000000000000711, 1.500000000000001332 ) ;
#10885=ORIENTED_EDGE ( 'NONE', *, *, #19620, .T. ) ;
#10886=CIRCLE ( 'NONE', #17158, 45.49665035954053138 ) ;
#10894=ORIENTED_EDGE ( 'NONE', *, *, #24975, .T. ) ;
#10896=FACE_OUTER_BOUND ( 'NONE', #2159, .T. ) ;
#10899=ORIENTED_EDGE ( 'NONE', *, *, #22375, .T. ) ;
#10901=AXIS2_PLACEMENT_3D ( 'NONE', #28643, #23718, #23073 ) ;
#10933=ORIENTED_EDGE ( 'NONE', *, *, #16837, .T. ) ;
#10938=VERTEX_POINT ( 'NONE', #26353 ) ;
#10947=CARTESIAN_POINT ( 'NONE',  ( 34.29950969015405349, 17.36467600858027183, 47.04930799450052348 ) ) ;
#10961=CIRCLE ( 'NONE', #15647, 46.67448298906162307 ) ;
#10963=ORIENTED_EDGE ( 'NONE', *, *, #8967, .T. ) ;
#10968=ORIENTED_EDGE ( 'NONE', *, *, #21322, .T. ) ;
#10983=DIRECTION ( 'NONE',  ( -1.000000000000000000, 0.000000000000000000, 0.000000000000000000 ) ) ;
#10990=ORIENTED_EDGE ( 'NONE', *, *, #30344, .T. ) ;
#11005=TOROIDAL_SURFACE ( 'NONE', #23034, 44.50000000000000000, 1.499999999999995115 ) ;
#11011=FACE_OUTER_BOUND ( 'NONE', #29600, .T. ) ;
#11015=DIRECTION ( 'NONE',  ( 0.000000000000000000, 0.000000000000000000, 1.000000000000000000 ) ) ;
#11023=DIRECTION ( 'NONE',  ( 1.000000000000000000, 0.000000000000000000, 0.000000000000000000 ) ) ;
#11025=EDGE_CURVE ( 'NONE', #27059, #22946, #19949, .T. ) ;
#11050=LINE ( 'NONE', #5801, #24390 ) ;
#11055=AXIS2_PLACEMENT_3D ( 'NONE', #159, #2463, #17883 ) ;
#11075=DIRECTION ( 'NONE',  ( -0.000000000000000000, -1.000000000000000000, 0.000000000000000000 ) ) ;
#11081=DIRECTION ( 'NONE',  ( -1.000000000000000000, 0.000000000000000000, 0.000000000000000000 ) ) ;
#11089=CLOSED_SHELL ( 'NONE', ( #11976, #12196, #20562, #16220, #16828, #23744, #4619, #29072, #27954, #25969, #30219, #20760, #9417, #12506, #2522, #7989, #3403, #12783, #25681, #29200, #7535, #13720, #17709, #29097, #2992, #30244, #18553, #10537, #19562, #2345, #14462, #19590, #10462, #20997, #31901, #13045, #2071, #20605, #11927, #19089, #9297, #21742, #23190, #9827, #14686, #17203, #616, #25687, #29656, #30678, #17631, #4072, #6750, #7242, #19866, #7952, #2182, #8370, #22852, #13284, #2407, #9536, #3970, #6630, #27886, #6046, #28671, #15971, #7033, #1432, #18334, #31296, #23639, #8780, #24987, #16346, #22936, #27269, #2193, #20488, #4375, #17062, #8930, #10449, #29351, #17776, #7542, #6350, #28133, #21149, #14971, #21186, #12825, #13020, #26451, #31306, #3443, #14355, #12543, #13359, #19448, #5420, #23130, #21598, #31756, #24229, #20199, #19401, #22566, #16039, #14244, #28309, #16475, #8232, #28529, #14274, #25796, #416 ) ) ;
#11098=CARTESIAN_POINT ( 'NONE',  ( 21.09785597605720753, -5.098646251524523443, 47.04930799450052348 ) ) ;
#11115=CARTESIAN_POINT ( 'NONE',  ( 46.59785597605721108, 13.86454579224779948, 47.04930799450052348 ) ) ;
#11122=AXIS2_PLACEMENT_3D ( 'NONE', #31450, #16333, #6656 ) ;
#11159=ORIENTED_EDGE ( 'NONE', *, *, #1245, .T. ) ;
#11163=AXIS2_PLACEMENT_3D ( 'NONE', #2938, #12968, #10983 ) ;
#11173=FACE_OUTER_BOUND ( 'NONE', #6082, .T. ) ;
#11176=LINE ( 'NONE', #23642, #28561 ) ;
#11182=AXIS2_PLACEMENT_3D ( 'NONE', #25070, #10142, #25238 ) ;
#11206=EDGE_LOOP ( 'NONE', ( #7983, #18087, #1212, #20499 ) ) ;
#11213=CARTESIAN_POINT ( 'NONE',  ( 7.282982007932096380, 15.57592086119046826, 47.04930799450052348 ) ) ;
#11214=DIRECTION ( 'NONE',  ( -1.000000000000000000, 0.000000000000000000, 0.000000000000000000 ) ) ;
#11215=CARTESIAN_POINT ( 'NONE',  ( 21.09785597605720753, 14.86454579224779948, 47.04930799450052348 ) ) ;
#11224=DIRECTION ( 'NONE',  ( -0.000000000000000000, -1.000000000000000000, 0.000000000000000000 ) ) ;
#11232=DIRECTION ( 'NONE',  ( -1.000000000000000000, 0.000000000000000000, 0.000000000000000000 ) ) ;
#11240=CYLINDRICAL_SURFACE ( 'NONE', #31398, 37.50000000000000711 ) ;
#11247=AXIS2_PLACEMENT_3D ( 'NONE', #3045, #20615, #12762 ) ;
#11251=ORIENTED_EDGE ( 'NONE', *, *, #6520, .F. ) ;
#11253=ORIENTED_EDGE ( 'NONE', *, *, #31267, .T. ) ;
#11261=DIRECTION ( 'NONE',  ( -0.000000000000000000, -1.000000000000000000, 0.000000000000000000 ) ) ;
#11264=ORIENTED_EDGE ( 'NONE', *, *, #21249, .F. ) ;
#11275=EDGE_CURVE ( 'NONE', #13490, #11782, #30951, .T. ) ;
#11301=CARTESIAN_POINT ( 'NONE',  ( 21.09785597605720753, 14.86454579224779948, 47.04930799450052348 ) ) ;
#11319=FACE_OUTER_BOUND ( 'NONE', #13195, .T. ) ;
#11329=VERTEX_POINT ( 'NONE', #30314 ) ;
#11371=SHAPE_REPRESENTATION ( 'Lower Suspension', ( #8172 ), #27017 ) ;
#11391=FACE_OUTER_BOUND ( 'NONE', #6417, .T. ) ;
#11398=AXIS2_PLACEMENT_3D ( 'NONE', #13341, #13498, #3791 ) ;
#11399=EDGE_CURVE ( 'NONE', #27481, #22149, #7410, .T. ) ;
#11402=DIRECTION ( 'NONE',  ( -1.000000000000000000, 0.000000000000000000, 0.000000000000000000 ) ) ;
#11431=CIRCLE ( 'NONE', #29786, 0.5000000000000004441 ) ;
#11434=EDGE_CURVE ( 'NONE', #19635, #19572, #30467, .T. ) ;
#11442=CARTESIAN_POINT ( 'NONE',  ( 21.09785597605720753, -5.098646251524523443, 47.04930799450052348 ) ) ;
#11478=CARTESIAN_POINT ( 'NONE',  ( 65.59785597605720397, 13.86454579224779948, 47.04930799450051637 ) ) ;
#11518=AXIS2_PLACEMENT_3D ( 'NONE', #14855, #20092, #233 ) ;
#11524=EDGE_CURVE ( 'NONE', #22190, #3892, #26018, .T. ) ;
#11525=CARTESIAN_POINT ( 'NONE',  ( -8.402144023942796025, 14.86454579224779948, 47.04930799450052348 ) ) ;
#11531=DIRECTION ( 'NONE',  ( -0.000000000000000000, -1.000000000000000000, 0.000000000000000000 ) ) ;
#11532=DIRECTION ( 'NONE',  ( -0.000000000000000000, -1.000000000000000000, 0.000000000000000000 ) ) ;
#11538=AXIS2_PLACEMENT_3D ( 'NONE', #1488, #13821, #16583 ) ;
#11543=CARTESIAN_POINT ( 'NONE',  ( -6.402144023942790696, 14.86454579224779948, 47.04930799450052348 ) ) ;
#11554=DIRECTION ( 'NONE',  ( -0.000000000000000000, -1.000000000000000000, 0.000000000000000000 ) ) ;
#11562=AXIS2_PLACEMENT_3D ( 'NONE', #28708, #3597, #21306 ) ;
#11575=CARTESIAN_POINT ( 'NONE',  ( 21.09785597605720753, -5.098646251524523443, 47.04930799450052348 ) ) ;
#11586=DIRECTION ( 'NONE',  ( -1.000000000000000000, 0.000000000000000000, 0.000000000000000000 ) ) ;
#11593=EDGE_LOOP ( 'NONE', ( #3869, #15169, #9580, #2677 ) ) ;
#11601=VECTOR ( 'NONE', #2003, 1000.000000000000000 ) ;
#11602=EDGE_CURVE ( 'NONE', #12393, #10938, #4183, .T. ) ;
#11616=CARTESIAN_POINT ( 'NONE',  ( 21.09785597605720753, 15.70210863493540288, 47.04930799450052348 ) ) ;
#11639=ORIENTED_EDGE ( 'NONE', *, *, #14026, .F. ) ;
#11643=ORIENTED_EDGE ( 'NONE', *, *, #28684, .T. ) ;
#11644=DIRECTION ( 'NONE',  ( -1.224646799147353207E-16, 0.000000000000000000, -1.000000000000000000 ) ) ;
#11652=DIRECTION ( 'NONE',  ( -1.000000000000000000, 0.000000000000000000, 0.000000000000000000 ) ) ;
#11671=DIRECTION ( 'NONE',  ( -0.000000000000000000, -1.000000000000000000, 0.000000000000000000 ) ) ;
#11712=DIRECTION ( 'NONE',  ( -1.000000000000000000, 0.000000000000000000, 0.000000000000000000 ) ) ;
#11720=DIRECTION ( 'NONE',  ( -0.000000000000000000, -1.000000000000000000, 0.000000000000000000 ) ) ;
#11727=AXIS2_PLACEMENT_3D ( 'NONE', #2546, #10273, #7972 ) ;
#11728=AXIS2_PLACEMENT_3D ( 'NONE', #6105, #16105, #30423 ) ;
#11729=AXIS2_PLACEMENT_3D ( 'NONE', #15390, #285, #3060 ) ;
#11735=DIRECTION ( 'NONE',  ( -0.000000000000000000, -1.000000000000000000, 0.000000000000000000 ) ) ;
#11737=CARTESIAN_POINT ( 'NONE',  ( 21.09785597605720753, 13.86454579224779948, 47.04930799450052348 ) ) ;
#11747=DIRECTION ( 'NONE',  ( -1.000000000000000000, 0.000000000000000000, 0.000000000000000000 ) ) ;
#11763=CIRCLE ( 'NONE', #12292, 0.1999999999999987899 ) ;
#11770=ORIENTED_EDGE ( 'NONE', *, *, #9200, .F. ) ;
#11773=LINE ( 'NONE', #7335, #21185 ) ;
#11782=VERTEX_POINT ( 'NONE', #27152 ) ;
#11799=CIRCLE ( 'NONE', #30149, 39.50000000000000000 ) ;
#11805=DIRECTION ( 'NONE',  ( -0.000000000000000000, -1.000000000000000000, 0.000000000000000000 ) ) ;
#11822=CARTESIAN_POINT ( 'NONE',  ( 21.09785597605720753, 14.56454579224780232, 47.04930799450052348 ) ) ;
#11841=DIRECTION ( 'NONE',  ( 1.000000000000000000, 0.000000000000000000, 0.000000000000000000 ) ) ;
#11847=EDGE_LOOP ( 'NONE', ( #2594, #16986, #22221, #11264 ) ) ;
#11874=ORIENTED_EDGE ( 'NONE', *, *, #30428, .T. ) ;
#11890=DIRECTION ( 'NONE',  ( -1.000000000000000000, 0.000000000000000000, 0.000000000000000000 ) ) ;
#11897=DIRECTION ( 'NONE',  ( -1.000000000000000000, 0.000000000000000000, 0.000000000000000000 ) ) ;
#11901=CARTESIAN_POINT ( 'NONE',  ( -17.40214402394279247, 13.86454579224779948, 47.04930799450052348 ) ) ;
#11903=DIRECTION ( 'NONE',  ( -0.000000000000000000, -1.000000000000000000, 0.000000000000000000 ) ) ;
#11909=DIRECTION ( 'NONE',  ( -1.000000000000000000, 0.000000000000000000, 0.000000000000000000 ) ) ;
#11925=ORIENTED_EDGE ( 'NONE', *, *, #5589, .F. ) ;
#11927=ADVANCED_FACE ( 'NONE', ( #30276 ), #25348, .F. ) ;
#11941=DIRECTION ( 'NONE',  ( -1.000000000000000000, 0.000000000000000000, 0.000000000000000000 ) ) ;
#11952=AXIS2_PLACEMENT_3D ( 'NONE', #26892, #14104, #16388 ) ;
#11958=EDGE_LOOP ( 'NONE', ( #6159, #20352, #21270, #4788 ) ) ;
#11966=ORIENTED_EDGE ( 'NONE', *, *, #4944, .F. ) ;
#11971=AXIS2_PLACEMENT_3D ( 'NONE', #24631, #22166, #31701 ) ;
#11975=CARTESIAN_POINT ( 'NONE',  ( 21.09785597605720753, -5.098646251524523443, 47.04930799450052348 ) ) ;
#11976=ADVANCED_FACE ( 'NONE', ( #26625 ), #1514, .T. ) ;
#11981=ORIENTED_EDGE ( 'NONE', *, *, #18374, .F. ) ;
#11985=TOROIDAL_SURFACE ( 'NONE', #26660, 17.50000000000000000, 1.999999999999998224 ) ;
#11993=DIRECTION ( 'NONE',  ( -0.000000000000000000, -1.000000000000000000, 0.000000000000000000 ) ) ;
#11995=CARTESIAN_POINT ( 'NONE',  ( 21.09785597605720753, 13.78276522714992147, 47.04930799450052348 ) ) ;
#12019=CARTESIAN_POINT ( 'NONE',  ( -22.40214402394279247, -5.098646251524523443, 47.04930799450052348 ) ) ;
#12069=ORIENTED_EDGE ( 'NONE', *, *, #8300, .F. ) ;
#12075=DIRECTION ( 'NONE',  ( -1.000000000000000000, 0.000000000000000000, 0.000000000000000000 ) ) ;
#12077=DIRECTION ( 'NONE',  ( -1.000000000000000000, 0.000000000000000000, 0.000000000000000000 ) ) ;
#12083=LINE ( 'NONE', #7151, #2535 ) ;
#12088=ORIENTED_EDGE ( 'NONE', *, *, #4536, .T. ) ;
#12092=AXIS2_PLACEMENT_3D ( 'NONE', #14343, #14671, #22034 ) ;
#12097=LINE ( 'NONE', #7819, #16666 ) ;
#12099=EDGE_LOOP ( 'NONE', ( #169, #11159, #21134, #2625 ) ) ;
#12104=DIRECTION ( 'NONE',  ( -0.000000000000000000, -1.000000000000000000, 0.000000000000000000 ) ) ;
#12116=DIRECTION ( 'NONE',  ( -1.000000000000000000, 0.000000000000000000, 0.000000000000000000 ) ) ;
#12129=DIRECTION ( 'NONE',  ( -1.000000000000000000, 0.000000000000000000, 0.000000000000000000 ) ) ;
#12135=AXIS2_PLACEMENT_3D ( 'NONE', #12742, #2868, #24876 ) ;
#12143=ORIENTED_EDGE ( 'NONE', *, *, #4300, .F. ) ;
#12159=VERTEX_POINT ( 'NONE', #20056 ) ;
#12182=CARTESIAN_POINT ( 'NONE',  ( 2.097855976057206639, 13.86454579224779948, 47.04930799450052348 ) ) ;
#12196=ADVANCED_FACE ( 'NONE', ( #9399 ), #15292, .T. ) ;
#12197=DIRECTION ( 'NONE',  ( -0.000000000000000000, -1.000000000000000000, 0.000000000000000000 ) ) ;
#12201=CARTESIAN_POINT ( 'NONE',  ( 48.59785597605720397, -5.098646251524523443, 47.04930799450052348 ) ) ;
#12207=ORIENTED_EDGE ( 'NONE', *, *, #3296, .F. ) ;
#12208=VERTEX_POINT ( 'NONE', #19723 ) ;
#12211=CARTESIAN_POINT ( 'NONE',  ( 7.896202261960366009, 17.36467600858027183, 47.04930799450052348 ) ) ;
#12212=DIRECTION ( 'NONE',  ( -0.000000000000000000, -1.000000000000000000, 0.000000000000000000 ) ) ;
#12244=EDGE_LOOP ( 'NONE', ( #4364, #26318, #23262, #9938 ) ) ;
#12255=CIRCLE ( 'NONE', #30597, 1.499999999999998668 ) ;
#12258=ORIENTED_EDGE ( 'NONE', *, *, #3982, .T. ) ;
#12266=CIRCLE ( 'NONE', #8079, 1.500000000000001332 ) ;
#12292=AXIS2_PLACEMENT_3D ( 'NONE', #380, #15639, #10576 ) ;
#12313=VERTEX_POINT ( 'NONE', #8007 ) ;
#12314=CARTESIAN_POINT ( 'NONE',  ( 67.09652168471781408, 13.80129159329807287, 47.04930799450051637 ) ) ;
#12318=EDGE_CURVE ( 'NONE', #29739, #15228, #7899, .T. ) ;
#12336=CIRCLE ( 'NONE', #7077, 46.67448298906162307 ) ;
#12337=AXIS2_PLACEMENT_3D ( 'NONE', #11901, #29632, #19269 ) ;
#12339=CIRCLE ( 'NONE', #3423, 40.00000000000000711 ) ;
#12354=DIRECTION ( 'NONE',  ( -0.000000000000000000, -1.000000000000000000, 0.000000000000000000 ) ) ;
#12372=DIRECTION ( 'NONE',  ( -1.224646799147353207E-16, 0.000000000000000000, -1.000000000000000000 ) ) ;
#12383=ORIENTED_EDGE ( 'NONE', *, *, #15247, .F. ) ;
#12387=AXIS2_PLACEMENT_3D ( 'NONE', #9855, #17716, #17227 ) ;
#12393=VERTEX_POINT ( 'NONE', #20630 ) ;
#12401=DIRECTION ( 'NONE',  ( -1.000000000000000000, 0.000000000000000000, 0.000000000000000000 ) ) ;
#12413=AXIS2_PLACEMENT_3D ( 'NONE', #2468, #9696, #20022 ) ;
#12428=DIRECTION ( 'NONE',  ( -0.000000000000000000, -1.000000000000000000, 0.000000000000000000 ) ) ;
#12433=EDGE_CURVE ( 'NONE', #15228, #29739, #29371, .T. ) ;
#12451=DIRECTION ( 'NONE',  ( -1.000000000000000000, 0.000000000000000000, 0.000000000000000000 ) ) ;
#12482=LINE ( 'NONE', #29712, #23711 ) ;
#12485=DIRECTION ( 'NONE',  ( 0.000000000000000000, 0.000000000000000000, 1.000000000000000000 ) ) ;
#12491=CARTESIAN_POINT ( 'NONE',  ( 7.596071960694295910, 17.16474120167318063, 47.04930799450052348 ) ) ;
#12494=ORIENTED_EDGE ( 'NONE', *, *, #25601, .F. ) ;
#12505=EDGE_LOOP ( 'NONE', ( #1933, #9989, #18682, #21118 ) ) ;
#12506=ADVANCED_FACE ( 'NONE', ( #2390 ), #5844, .T. ) ;
#12523=DIRECTION ( 'NONE',  ( -1.000000000000000000, 0.000000000000000000, 0.000000000000000000 ) ) ;
#12534=FACE_OUTER_BOUND ( 'NONE', #953, .T. ) ;
#12543=ADVANCED_FACE ( 'NONE', ( #17637 ), #5018, .F. ) ;
#12545=EDGE_CURVE ( 'NONE', #21091, #28622, #22051, .T. ) ;
#12603=DIRECTION ( 'NONE',  ( -1.000000000000000000, 0.000000000000000000, 0.000000000000000000 ) ) ;
#12607=AXIS2_PLACEMENT_3D ( 'NONE', #22800, #315, #30360 ) ;
#12633=DIRECTION ( 'NONE',  ( -1.000000000000000000, 0.000000000000000000, 0.000000000000000000 ) ) ;
#12644=DIRECTION ( 'NONE',  ( -0.000000000000000000, -1.000000000000000000, 0.000000000000000000 ) ) ;
#12647=EDGE_CURVE ( 'NONE', #24672, #23918, #15248, .T. ) ;
#12651=DIRECTION ( 'NONE',  ( -1.000000000000000000, 0.000000000000000000, 0.000000000000000000 ) ) ;
#12658=CYLINDRICAL_SURFACE ( 'NONE', #29817, 19.00000000000000000 ) ;
#12660=EDGE_CURVE ( 'NONE', #15228, #12910, #17868, .T. ) ;
#12680=AXIS2_PLACEMENT_3D ( 'NONE', #24539, #21907, #14378 ) ;
#12705=FACE_OUTER_BOUND ( 'NONE', #7313, .T. ) ;
#12706=CARTESIAN_POINT ( 'NONE',  ( -20.40214402394279603, 14.86454579224779948, 47.04930799450052348 ) ) ;
#12718=DIRECTION ( 'NONE',  ( 1.000000000000000000, 0.000000000000000000, 0.000000000000000000 ) ) ;
#12731=DIRECTION ( 'NONE',  ( -0.000000000000000000, -1.000000000000000000, 0.000000000000000000 ) ) ;
#12738=EDGE_CURVE ( 'NONE', #14305, #490, #31410, .T. ) ;
#12742=CARTESIAN_POINT ( 'NONE',  ( 34.59963999142011204, 15.70210863493540288, 47.04930799450052348 ) ) ;
#12762=DIRECTION ( 'NONE',  ( -1.000000000000000000, 0.000000000000000000, 0.000000000000000000 ) ) ;
#12778=EDGE_CURVE ( 'NONE', #12159, #16815, #23113, .T. ) ;
#12783=ADVANCED_FACE ( 'NONE', ( #31252 ), #29419, .T. ) ;
#12790=ORIENTED_EDGE ( 'NONE', *, *, #25283, .T. ) ;
#12804=VERTEX_POINT ( 'NONE', #1522 ) ;
#12812=DIRECTION ( 'NONE',  ( -1.000000000000000000, 0.000000000000000000, 0.000000000000000000 ) ) ;
#12820=DIRECTION ( 'NONE',  ( -1.000000000000000000, 0.000000000000000000, 0.000000000000000000 ) ) ;
#12822=VERTEX_POINT ( 'NONE', #11543 ) ;
#12825=ADVANCED_FACE ( 'NONE', ( #9080 ), #2690, .T. ) ;
#12859=CARTESIAN_POINT ( 'NONE',  ( 21.09785597605720753, 13.86454579224779948, 47.04930799450052348 ) ) ;
#12883=CIRCLE ( 'NONE', #31223, 1.500000000000001332 ) ;
#12885=STYLED_ITEM ( 'NONE', ( #4966 ), #4182 ) ;
#12910=VERTEX_POINT ( 'NONE', #7276 ) ;
#12912=CIRCLE ( 'NONE', #1332, 43.50000000000000000 ) ;
#12930=EDGE_LOOP ( 'NONE', ( #15436, #14366, #1415, #21697 ) ) ;
#12939=EDGE_LOOP ( 'NONE', ( #18038, #11874, #14607, #23833 ) ) ;
#12941=EDGE_LOOP ( 'NONE', ( #28655, #20949, #10933, #30758 ) ) ;
#12942=TOROIDAL_SURFACE ( 'NONE', #2954, 44.50000000000000000, 1.000000000000000000 ) ;
#12943=DIRECTION ( 'NONE',  ( -0.000000000000000000, -1.000000000000000000, 0.000000000000000000 ) ) ;
#12948=CIRCLE ( 'NONE', #9259, 21.50000000000000000 ) ;
#12957=ORIENTED_EDGE ( 'NONE', *, *, #5445, .T. ) ;
#12965=ORIENTED_EDGE ( 'NONE', *, *, #19998, .F. ) ;
#12968=DIRECTION ( 'NONE',  ( -0.000000000000000000, -1.000000000000000000, 0.000000000000000000 ) ) ;
#12970=DIRECTION ( 'NONE',  ( 1.000000000000000000, 0.000000000000000000, 0.000000000000000000 ) ) ;
#12972=ORIENTED_EDGE ( 'NONE', *, *, #20642, .T. ) ;
#12996=CIRCLE ( 'NONE', #30794, 27.49999999999998934 ) ;
#13005=DIRECTION ( 'NONE',  ( -0.000000000000000000, -1.000000000000000000, 0.000000000000000000 ) ) ;
#13006=CARTESIAN_POINT ( 'NONE',  ( -2.402144023942794249, 14.86454579224779948, 47.04930799450052348 ) ) ;
#13020=ADVANCED_FACE ( 'NONE', ( #16422 ), #4653, .F. ) ;
#13037=CONICAL_SURFACE ( 'NONE', #23503, 15.23374605753642186, 1.187672012580060610 ) ;
#13038=AXIS2_PLACEMENT_3D ( 'NONE', #2652, #20207, #27924 ) ;
#13045=ADVANCED_FACE ( 'NONE', ( #1483 ), #11985, .T. ) ;
#13098=DIRECTION ( 'NONE',  ( -1.000000000000000000, 0.000000000000000000, 0.000000000000000000 ) ) ;
#13123=CIRCLE ( 'NONE', #15278, 25.00000000000000000 ) ;
#13139=DIRECTION ( 'NONE',  ( -0.000000000000000000, -1.000000000000000000, 0.000000000000000000 ) ) ;
#13165=FACE_OUTER_BOUND ( 'NONE', #26662, .T. ) ;
#13168=AXIS2_PLACEMENT_3D ( 'NONE', #25910, #8833, #30848 ) ;
#13192=CIRCLE ( 'NONE', #22086, 46.09082119073493544 ) ;
#13195=EDGE_LOOP ( 'NONE', ( #18318, #17304, #10575, #13457 ) ) ;
#13202=VECTOR ( 'NONE', #11261, 1000.000000000000000 ) ;
#13203=CARTESIAN_POINT ( 'NONE',  ( 21.09785597605720753, 14.66454579224780019, 47.04930799450052348 ) ) ;
#13206=CIRCLE ( 'NONE', #11122, 24.99999999999999645 ) ;
#13219=CARTESIAN_POINT ( 'NONE',  ( 21.09785597605720753, 13.86454579224779948, 47.04930799450052348 ) ) ;
#13222=EDGE_LOOP ( 'NONE', ( #30783, #10968, #8506, #24020 ) ) ;
#13223=CONICAL_SURFACE ( 'NONE', #3244, 15.23374605753642186, 1.187672012580060610 ) ;
#13235=VERTEX_POINT ( 'NONE', #29722 ) ;
#13239=EDGE_CURVE ( 'NONE', #665, #2312, #19326, .T. ) ;
#13271=CARTESIAN_POINT ( 'NONE',  ( 21.09785597605720753, 13.86454579224779948, 47.04930799450052348 ) ) ;
#13275=EDGE_LOOP ( 'NONE', ( #16629, #5188, #4325, #7697 ) ) ;
#13284=ADVANCED_FACE ( 'NONE', ( #2309, #22322 ), #20829, .F. ) ;
#13286=EDGE_CURVE ( 'NONE', #22149, #30896, #7817, .T. ) ;
#13297=FACE_OUTER_BOUND ( 'NONE', #19924, .T. ) ;
#13298=FACE_OUTER_BOUND ( 'NONE', #29901, .T. ) ;
#13301=CARTESIAN_POINT ( 'NONE',  ( -21.90214402394279603, 13.86454579224779948, 47.04930799450052348 ) ) ;
#13303=CARTESIAN_POINT ( 'NONE',  ( 21.09785597605720753, 13.68462854903246573, 47.04930799450052348 ) ) ;
#13341=CARTESIAN_POINT ( 'NONE',  ( 21.09785597605720753, 14.86454579224779948, 47.04930799450052348 ) ) ;
#13355=ORIENTED_EDGE ( 'NONE', *, *, #31507, .T. ) ;
#13359=ADVANCED_FACE ( 'NONE', ( #8208 ), #22488, .T. ) ;
#13364=VERTEX_POINT ( 'NONE', #10514 ) ;
#13373=TOROIDAL_SURFACE ( 'NONE', #22248, 13.50178401536290806, 0.5000000000000002220 ) ;
#13374=CIRCLE ( 'NONE', #19623, 19.50000000000000000 ) ;
#13380=DIRECTION ( 'NONE',  ( -1.000000000000000000, 0.000000000000000000, 0.000000000000000000 ) ) ;
#13398=EDGE_CURVE ( 'NONE', #17663, #26196, #20919, .T. ) ;
#13406=DIRECTION ( 'NONE',  ( -1.000000000000000000, 0.000000000000000000, 0.000000000000000000 ) ) ;
#13408=DIRECTION ( 'NONE',  ( -1.000000000000000000, 0.000000000000000000, 0.000000000000000000 ) ) ;
#13422=LINE ( 'NONE', #30813, #4910 ) ;
#13424=DIRECTION ( 'NONE',  ( -1.000000000000000000, 0.000000000000000000, 0.000000000000000000 ) ) ;
#13440=CIRCLE ( 'NONE', #17616, 13.00178401536290806 ) ;
#13443=DIRECTION ( 'NONE',  ( 0.000000000000000000, 0.000000000000000000, 1.000000000000000000 ) ) ;
#13450=TOROIDAL_SURFACE ( 'NONE', #17081, 29.50000000000000355, 1.500000000000001332 ) ;
#13454=DIRECTION ( 'NONE',  ( -0.000000000000000000, -1.000000000000000000, 0.000000000000000000 ) ) ;
#13457=ORIENTED_EDGE ( 'NONE', *, *, #11602, .F. ) ;
#13474=DIRECTION ( 'NONE',  ( 1.000000000000000000, 0.000000000000000000, 0.000000000000000000 ) ) ;
#13479=DIRECTION ( 'NONE',  ( -1.000000000000000000, 0.000000000000000000, 0.000000000000000000 ) ) ;
#13490=VERTEX_POINT ( 'NONE', #3431 ) ;
#13498=DIRECTION ( 'NONE',  ( -0.000000000000000000, -1.000000000000000000, 0.000000000000000000 ) ) ;
#13514=CARTESIAN_POINT ( 'NONE',  ( -6.902144023942794249, 14.86454579224779948, 47.04930799450052348 ) ) ;
#13558=CARTESIAN_POINT ( 'NONE',  ( 55.09785597605721108, -5.098646251524523443, 47.04930799450051637 ) ) ;
#13577=AXIS2_PLACEMENT_3D ( 'NONE', #5511, #2876, #30296 ) ;
#13580=EDGE_CURVE ( 'NONE', #22946, #9753, #15170, .T. ) ;
#13599=VERTEX_POINT ( 'NONE', #9823 ) ;
#13608=DIRECTION ( 'NONE',  ( -1.000000000000000000, 0.000000000000000000, 0.000000000000000000 ) ) ;
#13612=CARTESIAN_POINT ( 'NONE',  ( 21.09785597605720753, 13.86454579224779948, 47.04930799450052348 ) ) ;
#13634=ORIENTED_EDGE ( 'NONE', *, *, #18846, .F. ) ;
#13642=EDGE_CURVE ( 'NONE', #26091, #22946, #1206, .T. ) ;
#13676=CIRCLE ( 'NONE', #26782, 37.00000000000000711 ) ;
#13683=CARTESIAN_POINT ( 'NONE',  ( 54.59785597605721108, 14.86454579224779948, 47.04930799450051637 ) ) ;
#13693=DIRECTION ( 'NONE',  ( 1.000000000000000000, 0.000000000000000000, 0.000000000000000000 ) ) ;
#13696=DIRECTION ( 'NONE',  ( -0.000000000000000000, -1.000000000000000000, 0.000000000000000000 ) ) ;
#13702=CARTESIAN_POINT ( 'NONE',  ( 21.09785597605720753, 13.86454579224779948, 47.04930799450052348 ) ) ;
#13708=CIRCLE ( 'NONE', #14758, 15.23374605753642186 ) ;
#13720=ADVANCED_FACE ( 'NONE', ( #10605 ), #14662, .T. ) ;
#13754=EDGE_CURVE ( 'NONE', #12313, #13235, #24083, .T. ) ;
#13770=DIRECTION ( 'NONE',  ( -1.000000000000000000, 0.000000000000000000, 0.000000000000000000 ) ) ;
#13786=TOROIDAL_SURFACE ( 'NONE', #11163, 46.39830989763677849, 0.4000000000000020206 ) ;
#13796=DIRECTION ( 'NONE',  ( -0.000000000000000000, -1.000000000000000000, 0.000000000000000000 ) ) ;
#13813=DIRECTION ( 'NONE',  ( -1.000000000000000000, 0.000000000000000000, 0.000000000000000000 ) ) ;
#13821=DIRECTION ( 'NONE',  ( -1.224646799147353207E-16, 0.000000000000000000, -1.000000000000000000 ) ) ;
#13824=DIRECTION ( 'NONE',  ( -1.000000000000000000, 0.000000000000000000, 0.000000000000000000 ) ) ;
#13827=ORIENTED_EDGE ( 'NONE', *, *, #18576, .T. ) ;
#13848=CARTESIAN_POINT ( 'NONE',  ( 21.09785597605720753, 16.03967147762301693, 47.04930799450052348 ) ) ;
#13851=CARTESIAN_POINT ( 'NONE',  ( 21.09785597605720753, 14.66454579224779842, 47.04930799450052348 ) ) ;
#13877=ORIENTED_EDGE ( 'NONE', *, *, #29680, .T. ) ;
#13880=AXIS2_PLACEMENT_3D ( 'NONE', #16557, #26575, #11652 ) ;
#13892=DIRECTION ( 'NONE',  ( -1.224646799147353207E-16, 0.000000000000000000, -1.000000000000000000 ) ) ;
#13911=ORIENTED_EDGE ( 'NONE', *, *, #31875, .T. ) ;
#13916=FACE_OUTER_BOUND ( 'NONE', #27284, .T. ) ;
#13945=VERTEX_POINT ( 'NONE', #29444 ) ;
#13946=DIRECTION ( 'NONE',  ( -1.000000000000000000, 0.000000000000000000, 0.000000000000000000 ) ) ;
#13948=EDGE_CURVE ( 'NONE', #1796, #21091, #15198, .T. ) ;
#13955=ORIENTED_EDGE ( 'NONE', *, *, #12660, .T. ) ;
#13957=DIRECTION ( 'NONE',  ( -0.000000000000000000, -1.000000000000000000, 0.000000000000000000 ) ) ;
#13959=AXIS2_PLACEMENT_3D ( 'NONE', #27143, #9762, #27317 ) ;
#13961=DIRECTION ( 'NONE',  ( -1.000000000000000000, 0.000000000000000000, 0.000000000000000000 ) ) ;
#13975=AXIS2_PLACEMENT_3D ( 'NONE', #13612, #8206, #23617 ) ;
#13996=ORIENTED_EDGE ( 'NONE', *, *, #6859, .F. ) ;
#13998=CARTESIAN_POINT ( 'NONE',  ( -33.00214402394279745, 14.66454579224780019, 47.04930799450052348 ) ) ;
#14015=CYLINDRICAL_SURFACE ( 'NONE', #7863, 22.00000000000000000 ) ;
#14021=DIRECTION ( 'NONE',  ( -0.000000000000000000, -1.000000000000000000, 0.000000000000000000 ) ) ;
#14026=EDGE_CURVE ( 'NONE', #22237, #13235, #14673, .T. ) ;
#14028=EDGE_CURVE ( 'NONE', #29883, #2441, #22207, .T. ) ;
#14047=ORIENTED_EDGE ( 'NONE', *, *, #161, .F. ) ;
#14095=DIRECTION ( 'NONE',  ( -1.000000000000000000, 0.000000000000000000, 0.000000000000000000 ) ) ;
#14104=DIRECTION ( 'NONE',  ( -0.000000000000000000, -1.000000000000000000, 0.000000000000000000 ) ) ;
#14110=AXIS2_PLACEMENT_3D ( 'NONE', #17281, #1867, #19418 ) ;
#14114=AXIS2_PLACEMENT_3D ( 'NONE', #11995, #7, #24788 ) ;
#14118=DIRECTION ( 'NONE',  ( -0.000000000000000000, -1.000000000000000000, 0.000000000000000000 ) ) ;
#14167=CIRCLE ( 'NONE', #27254, 25.50000000000000355 ) ;
#14172=( LENGTH_UNIT ( ) NAMED_UNIT ( * ) SI_UNIT ( .MILLI., .METRE. ) );
#14181=DIRECTION ( 'NONE',  ( -1.000000000000000000, 0.000000000000000000, 0.000000000000000000 ) ) ;
#14206=ORIENTED_EDGE ( 'NONE', *, *, #28098, .F. ) ;
#14218=CARTESIAN_POINT ( 'NONE',  ( 43.09785597605720397, -5.098646251524523443, 47.04930799450052348 ) ) ;
#14220=VECTOR ( 'NONE', #13454, 1000.000000000000000 ) ;
#14225=AXIS2_PLACEMENT_3D ( 'NONE', #32102, #29967, #15183 ) ;
#14244=ADVANCED_FACE ( 'NONE', ( #18061 ), #28408, .F. ) ;
#14263=CIRCLE ( 'NONE', #1664, 45.99866570866061011 ) ;
#14264=DIRECTION ( 'NONE',  ( -0.000000000000000000, -1.000000000000000000, 0.000000000000000000 ) ) ;
#14270=EDGE_CURVE ( 'NONE', #25938, #25493, #23060, .T. ) ;
#14272=DIRECTION ( 'NONE',  ( -1.224646799147353207E-16, 0.000000000000000000, -1.000000000000000000 ) ) ;
#14273=CYLINDRICAL_SURFACE ( 'NONE', #21419, 43.50000000000000000 ) ;
#14274=ADVANCED_FACE ( 'NONE', ( #10853, #11011 ), #20842, .F. ) ;
#14281=DIRECTION ( 'NONE',  ( -1.000000000000000000, 0.000000000000000000, 0.000000000000000000 ) ) ;
#14282=TOROIDAL_SURFACE ( 'NONE', #5898, 35.50000000000000711, 2.000000000000001776 ) ;
#14284=DIRECTION ( 'NONE',  ( -1.224646799147353207E-16, 0.000000000000000000, -1.000000000000000000 ) ) ;
#14288=ORIENTED_EDGE ( 'NONE', *, *, #21993, .F. ) ;
#14303=CIRCLE ( 'NONE', #144, 27.49999999999998934 ) ;
#14305=VERTEX_POINT ( 'NONE', #19343 ) ;
#14306=CARTESIAN_POINT ( 'NONE',  ( -11.40214402394279603, 13.86454579224779948, 47.04930799450052348 ) ) ;
#14343=CARTESIAN_POINT ( 'NONE',  ( 21.09785597605720753, 14.86454579224779948, 47.04930799450052348 ) ) ;
#14344=DIRECTION ( 'NONE',  ( -1.000000000000000000, 0.000000000000000000, 0.000000000000000000 ) ) ;
#14354=EDGE_CURVE ( 'NONE', #19168, #17364, #29045, .T. ) ;
#14355=ADVANCED_FACE ( 'NONE', ( #11173 ), #23595, .F. ) ;
#14357=CIRCLE ( 'NONE', #20631, 22.00000000000000000 ) ;
#14366=ORIENTED_EDGE ( 'NONE', *, *, #28074, .T. ) ;
#14368=DIRECTION ( 'NONE',  ( -0.000000000000000000, -1.000000000000000000, 0.000000000000000000 ) ) ;
#14378=DIRECTION ( 'NONE',  ( -1.000000000000000000, 0.000000000000000000, 0.000000000000000000 ) ) ;
#14385=ORIENTED_EDGE ( 'NONE', *, *, #6410, .F. ) ;
#14386=UNCERTAINTY_MEASURE_WITH_UNIT (LENGTH_MEASURE( 1.000000000000000082E-05 ), #27772, 'distance_accuracy_value', 'NONE');
#14391=CIRCLE ( 'NONE', #18057, 24.99999999999999645 ) ;
#14404=DIRECTION ( 'NONE',  ( -1.000000000000000000, 0.000000000000000000, 0.000000000000000000 ) ) ;
#14407=ORIENTED_EDGE ( 'NONE', *, *, #5496, .F. ) ;
#14412=DIRECTION ( 'NONE',  ( -1.224646799147353207E-16, 0.000000000000000000, -1.000000000000000000 ) ) ;
#14422=AXIS2_PLACEMENT_3D ( 'NONE', #7510, #7671, #7997 ) ;
#14450=ORIENTED_EDGE ( 'NONE', *, *, #20038, .T. ) ;
#14462=ADVANCED_FACE ( 'NONE', ( #27672 ), #2112, .T. ) ;
#14469=ORIENTED_EDGE ( 'NONE', *, *, #13580, .F. ) ;
#14486=AXIS2_PLACEMENT_3D ( 'NONE', #30732, #1159, #28583 ) ;
#14492=CARTESIAN_POINT ( 'NONE',  ( -6.402144023942787143, -5.098646251524523443, 47.04930799450052348 ) ) ;
#14505=CARTESIAN_POINT ( 'NONE',  ( 21.09785597605720753, -5.098646251524523443, 47.04930799450052348 ) ) ;
#14511=CARTESIAN_POINT ( 'NONE',  ( 40.59785597605721108, -5.098646251524523443, 47.04930799450052348 ) ) ;
#14525=ORIENTED_EDGE ( 'NONE', *, *, #4346, .T. ) ;
#14532=CIRCLE ( 'NONE', #7198, 54.30000000000000426 ) ;
#14544=CARTESIAN_POINT ( 'NONE',  ( 40.59785597605721108, 14.86454579224779948, 47.04930799450052348 ) ) ;
#14557=CYLINDRICAL_SURFACE ( 'NONE', #15075, 54.30000000000000426 ) ;
#14559=CARTESIAN_POINT ( 'NONE',  ( 21.09785597605720753, 13.61454579224779771, 47.04930799450052348 ) ) ;
#14562=ORIENTED_EDGE ( 'NONE', *, *, #4038, .T. ) ;
#14571=DIRECTION ( 'NONE',  ( -1.000000000000000000, 0.000000000000000000, 0.000000000000000000 ) ) ;
#14577=CARTESIAN_POINT ( 'NONE',  ( 21.09785597605720753, -5.098646251524523443, 47.04930799450052348 ) ) ;
#14583=VECTOR ( 'NONE', #32446, 1000.000000000000000 ) ;
#14600=AXIS2_PLACEMENT_3D ( 'NONE', #31341, #8531, #16070 ) ;
#14602=VECTOR ( 'NONE', #6582, 1000.000000000000000 ) ;
#14607=ORIENTED_EDGE ( 'NONE', *, *, #1815, .T. ) ;
#14620=CARTESIAN_POINT ( 'NONE',  ( 67.63274615763145903, 14.86454579224779948, 47.04930799450051637 ) ) ;
#14639=DIRECTION ( 'NONE',  ( 1.000000000000000000, 0.000000000000000000, 0.000000000000000000 ) ) ;
#14662=TOROIDAL_SURFACE ( 'NONE', #21966, 20.49999999999999645, 1.499999999999997780 ) ;
#14666=AXIS2_PLACEMENT_3D ( 'NONE', #31983, #11805, #21800 ) ;
#14671=DIRECTION ( 'NONE',  ( -0.000000000000000000, -1.000000000000000000, 0.000000000000000000 ) ) ;
#14673=LINE ( 'NONE', #12211, #30410 ) ;
#14686=ADVANCED_FACE ( 'NONE', ( #21725 ), #1543, .T. ) ;
#14693=ORIENTED_EDGE ( 'NONE', *, *, #19747, .F. ) ;
#14711=ORIENTED_EDGE ( 'NONE', *, *, #28441, .T. ) ;
#14717=ORIENTED_EDGE ( 'NONE', *, *, #5589, .T. ) ;
#14720=EDGE_CURVE ( 'NONE', #22190, #13364, #29241, .T. ) ;
#14724=FACE_OUTER_BOUND ( 'NONE', #26311, .T. ) ;
#14727=FACE_OUTER_BOUND ( 'NONE', #12941, .T. ) ;
#14758=AXIS2_PLACEMENT_3D ( 'NONE', #18945, #28816, #4355 ) ;
#14778=AXIS2_PLACEMENT_3D ( 'NONE', #23563, #8480, #3052 ) ;
#14797=CIRCLE ( 'NONE', #1160, 13.00178401536290806 ) ;
#14809=EDGE_LOOP ( 'NONE', ( #18785, #7416, #18139, #20035 ) ) ;
#14814=CARTESIAN_POINT ( 'NONE',  ( 21.09785597605720753, 13.86454579224779948, 47.04930799450052348 ) ) ;
#14832=CARTESIAN_POINT ( 'NONE',  ( 50.59785597605720397, 14.86454579224779948, 47.04930799450051637 ) ) ;
#14841=DIRECTION ( 'NONE',  ( -0.9999997877697283100, 0.0006515063303658816165, -1.224646539240230088E-16 ) ) ;
#14852=ORIENTED_EDGE ( 'NONE', *, *, #29084, .T. ) ;
#14855=CARTESIAN_POINT ( 'NONE',  ( 35.09963999142011204, 16.03967147762300982, 47.04930799450052348 ) ) ;
#14876=AXIS2_PLACEMENT_3D ( 'NONE', #28152, #15987, #30617 ) ;
#14895=ORIENTED_EDGE ( 'NONE', *, *, #18040, .T. ) ;
#14904=CARTESIAN_POINT ( 'NONE',  ( 21.09785597605720753, 13.86454579224779948, 47.04930799450052348 ) ) ;
#14925=CARTESIAN_POINT ( 'NONE',  ( 21.09785597605720753, -5.098646251524523443, 47.04930799450052348 ) ) ;
#14957=CYLINDRICAL_SURFACE ( 'NONE', #22777, 34.00000000000000000 ) ;
#14971=ADVANCED_FACE ( 'NONE', ( #23681 ), #24535, .T. ) ;
#14991=ORIENTED_EDGE ( 'NONE', *, *, #31836, .F. ) ;
#14993=DIRECTION ( 'NONE',  ( 1.000000000000000000, 0.000000000000000000, 0.000000000000000000 ) ) ;
#15004=ORIENTED_EDGE ( 'NONE', *, *, #9122, .F. ) ;
#15027=CARTESIAN_POINT ( 'NONE',  ( 21.09785597605720753, 13.86454579224779948, 47.04930799450052348 ) ) ;
#15029=DIRECTION ( 'NONE',  ( -1.000000000000000000, 0.000000000000000000, 0.000000000000000000 ) ) ;
#15041=EDGE_CURVE ( 'NONE', #10620, #25220, #8302, .T. ) ;
#15047=EDGE_LOOP ( 'NONE', ( #1433, #30132, #1762, #29658 ) ) ;
#15051=CARTESIAN_POINT ( 'NONE',  ( 21.09785597605720753, 13.86454579224779948, 47.04930799450052348 ) ) ;
#15052=DIRECTION ( 'NONE',  ( -0.000000000000000000, -1.000000000000000000, 0.000000000000000000 ) ) ;
#15055=EDGE_LOOP ( 'NONE', ( #13355, #28167, #2691, #30308 ) ) ;
#15058=VERTEX_POINT ( 'NONE', #18899 ) ;
#15068=ORIENTED_EDGE ( 'NONE', *, *, #12738, .T. ) ;
#15075=AXIS2_PLACEMENT_3D ( 'NONE', #29324, #26540, #21926 ) ;
#15082=ORIENTED_EDGE ( 'NONE', *, *, #6150, .F. ) ;
#15121=ORIENTED_EDGE ( 'NONE', *, *, #19747, .T. ) ;
#15133=CARTESIAN_POINT ( 'NONE',  ( 52.09785597605720397, 14.86454579224779948, 47.04930799450051637 ) ) ;
#15138=DIRECTION ( 'NONE',  ( -0.000000000000000000, -1.000000000000000000, 0.000000000000000000 ) ) ;
#15140=ORIENTED_EDGE ( 'NONE', *, *, #29493, .T. ) ;
#15149=DIRECTION ( 'NONE',  ( -1.000000000000000000, 0.000000000000000000, 0.000000000000000000 ) ) ;
#15150=DIRECTION ( 'NONE',  ( -1.000000000000000000, 0.000000000000000000, 0.000000000000000000 ) ) ;
#15169=ORIENTED_EDGE ( 'NONE', *, *, #2311, .T. ) ;
#15170=CIRCLE ( 'NONE', #3609, 37.50000000000000711 ) ;
#15177=CARTESIAN_POINT ( 'NONE',  ( 21.09785597605720753, 13.86454579224779948, 47.04930799450052348 ) ) ;
#15183=DIRECTION ( 'NONE',  ( -1.000000000000000000, 0.000000000000000000, 0.000000000000000000 ) ) ;
#15198=CIRCLE ( 'NONE', #29338, 16.00569570871410008 ) ;
#15228=VERTEX_POINT ( 'NONE', #22830 ) ;
#15231=DIRECTION ( 'NONE',  ( -0.000000000000000000, -1.000000000000000000, 0.000000000000000000 ) ) ;
#15247=EDGE_CURVE ( 'NONE', #17931, #23918, #10367, .T. ) ;
#15248=CIRCLE ( 'NONE', #581, 13.00178401536290806 ) ;
#15254=ORIENTED_EDGE ( 'NONE', *, *, #5274, .T. ) ;
#15255=DIRECTION ( 'NONE',  ( -1.000000000000000000, 0.000000000000000000, 0.000000000000000000 ) ) ;
#15261=DIRECTION ( 'NONE',  ( -0.000000000000000000, -1.000000000000000000, 0.000000000000000000 ) ) ;
#15278=AXIS2_PLACEMENT_3D ( 'NONE', #9812, #22271, #19974 ) ;
#15283=ORIENTED_EDGE ( 'NONE', *, *, #18, .F. ) ;
#15289=CIRCLE ( 'NONE', #22619, 1.500000000000001332 ) ;
#15290=DIRECTION ( 'NONE',  ( -0.000000000000000000, -1.000000000000000000, 0.000000000000000000 ) ) ;
#15292=TOROIDAL_SURFACE ( 'NONE', #23673, 54.10000000000000142, 0.1999999999999994282 ) ;
#15304=EDGE_LOOP ( 'NONE', ( #16226, #5532, #164, #21882 ) ) ;
#15327=CARTESIAN_POINT ( 'NONE',  ( 21.09785597605720753, 13.61454579224779771, 47.04930799450052348 ) ) ;
#15335=DIRECTION ( 'NONE',  ( -1.224646799147353207E-16, 0.000000000000000000, -1.000000000000000000 ) ) ;
#15345=EDGE_LOOP ( 'NONE', ( #28180, #13911, #1835, #27166 ) ) ;
#15361=EDGE_CURVE ( 'NONE', #10568, #23541, #14303, .T. ) ;
#15363=ORIENTED_EDGE ( 'NONE', *, *, #28402, .F. ) ;
#15387=AXIS2_PLACEMENT_3D ( 'NONE', #7117, #61, #30105 ) ;
#15390=CARTESIAN_POINT ( 'NONE',  ( 21.09785597605720753, 13.86454579224779948, 47.04930799450052348 ) ) ;
#15393=ORIENTED_EDGE ( 'NONE', *, *, #28684, .F. ) ;
#15430=CARTESIAN_POINT ( 'NONE',  ( -0.9021440239427910290, 13.86454579224779948, 47.04930799450052348 ) ) ;
#15436=ORIENTED_EDGE ( 'NONE', *, *, #13239, .F. ) ;
#15441=CIRCLE ( 'NONE', #14422, 54.10000000000000142 ) ;
#15453=EDGE_CURVE ( 'NONE', #18652, #28622, #22163, .T. ) ;
#15454=LINE ( 'NONE', #17258, #9094 ) ;
#15457=CYLINDRICAL_SURFACE ( 'NONE', #1573, 39.49999999999999289 ) ;
#15475=AXIS2_PLACEMENT_3D ( 'NONE', #16816, #26838, #4354 ) ;
#15479=CIRCLE ( 'NONE', #13880, 19.50000000000000000 ) ;
#15490=AXIS2_PLACEMENT_3D ( 'NONE', #15177, #12731, #27817 ) ;
#15497=LINE ( 'NONE', #25824, #20958 ) ;
#15506=DIRECTION ( 'NONE',  ( 1.000000000000000000, 0.000000000000000000, 0.000000000000000000 ) ) ;
#15519=VERTEX_POINT ( 'NONE', #18860 ) ;
#15533=ORIENTED_EDGE ( 'NONE', *, *, #9626, .F. ) ;
#15556=TOROIDAL_SURFACE ( 'NONE', #31299, 13.30178401536290878, 0.2000000000000002609 ) ;
#15562=DIRECTION ( 'NONE',  ( 1.000000000000000000, 0.000000000000000000, 0.000000000000000000 ) ) ;
#15576=DIRECTION ( 'NONE',  ( -1.000000000000000000, 0.000000000000000000, 0.000000000000000000 ) ) ;
#15579=DIRECTION ( 'NONE',  ( -1.000000000000000000, 0.000000000000000000, 0.000000000000000000 ) ) ;
#15583=DIRECTION ( 'NONE',  ( -0.000000000000000000, -1.000000000000000000, 0.000000000000000000 ) ) ;
#15590=ORIENTED_EDGE ( 'NONE', *, *, #31273, .F. ) ;
#15612=ORIENTED_EDGE ( 'NONE', *, *, #7768, .T. ) ;
#15639=DIRECTION ( 'NONE',  ( 0.000000000000000000, 0.000000000000000000, 1.000000000000000000 ) ) ;
#15640=DIRECTION ( 'NONE',  ( -1.000000000000000000, 0.000000000000000000, 0.000000000000000000 ) ) ;
#15647=AXIS2_PLACEMENT_3D ( 'NONE', #21019, #16256, #1482 ) ;
#15648=DIRECTION ( 'NONE',  ( -1.000000000000000000, 0.000000000000000000, 0.000000000000000000 ) ) ;
#15650=CARTESIAN_POINT ( 'NONE',  ( 21.09785597605720753, -5.098646251524523443, 47.04930799450052348 ) ) ;
#15655=DIRECTION ( 'NONE',  ( 1.000000000000000000, 0.000000000000000000, 0.000000000000000000 ) ) ;
#15660=DIRECTION ( 'NONE',  ( -0.000000000000000000, -1.000000000000000000, 0.000000000000000000 ) ) ;
#15667=DIRECTION ( 'NONE',  ( -1.000000000000000000, 0.000000000000000000, 0.000000000000000000 ) ) ;
#15684=CARTESIAN_POINT ( 'NONE',  ( 21.09785597605720753, 14.46497581658974063, 47.04930799450052348 ) ) ;
#15701=DIRECTION ( 'NONE',  ( -0.000000000000000000, -1.000000000000000000, 0.000000000000000000 ) ) ;
#15711=CARTESIAN_POINT ( 'NONE',  ( -18.40214402394278892, -5.098646251524523443, 47.04930799450052348 ) ) ;
#15721=AXIS2_PLACEMENT_3D ( 'NONE', #2242, #12428, #18105 ) ;
#15722=VERTEX_POINT ( 'NONE', #15898 ) ;
#15724=AXIS2_PLACEMENT_3D ( 'NONE', #5899, #15905, #2782 ) ;
#15739=DIRECTION ( 'NONE',  ( 0.000000000000000000, 0.000000000000000000, 1.000000000000000000 ) ) ;
#15745=CARTESIAN_POINT ( 'NONE',  ( -33.20214402394279318, 14.56454579224780232, 47.04930799450052348 ) ) ;
#15747=DIRECTION ( 'NONE',  ( 1.000000000000000000, 0.000000000000000000, 0.000000000000000000 ) ) ;
#15748=DIRECTION ( 'NONE',  ( -1.000000000000000000, 0.000000000000000000, 0.000000000000000000 ) ) ;
#15752=FACE_OUTER_BOUND ( 'NONE', #4207, .T. ) ;
#15769=CIRCLE ( 'NONE', #21509, 54.10000000000000142 ) ;
#15779=TOROIDAL_SURFACE ( 'NONE', #13168, 23.50000000000000000, 1.500000000000001332 ) ;
#15810=VERTEX_POINT ( 'NONE', #9144 ) ;
#15825=CARTESIAN_POINT ( 'NONE',  ( 21.09785597605720753, 14.56454579224780055, 47.04930799450052348 ) ) ;
#15832=CARTESIAN_POINT ( 'NONE',  ( 44.59785597605720397, 14.86454579224779948, 47.04930799450052348 ) ) ;
#15834=CARTESIAN_POINT ( 'NONE',  ( 21.09785597605720753, 13.86454579224779948, 47.04930799450052348 ) ) ;
#15852=DIRECTION ( 'NONE',  ( -1.224646799147353207E-16, 0.000000000000000000, -1.000000000000000000 ) ) ;
#15889=AXIS2_PLACEMENT_3D ( 'NONE', #17507, #24899, #2568 ) ;
#15898=CARTESIAN_POINT ( 'NONE',  ( 54.59785597605721108, 13.86454579224779948, 47.04930799450051637 ) ) ;
#15905=DIRECTION ( 'NONE',  ( -0.000000000000000000, -1.000000000000000000, 0.000000000000000000 ) ) ;
#15916=DIRECTION ( 'NONE',  ( -1.000000000000000000, 0.000000000000000000, 0.000000000000000000 ) ) ;
#15942=ORIENTED_EDGE ( 'NONE', *, *, #3110, .F. ) ;
#15952=AXIS2_PLACEMENT_3D ( 'NONE', #11525, #24317, #19056 ) ;
#15971=ADVANCED_FACE ( 'NONE', ( #29662 ), #23748, .F. ) ;
#15976=EDGE_LOOP ( 'NONE', ( #12383, #12494, #30829, #21008 ) ) ;
#15987=DIRECTION ( 'NONE',  ( -0.000000000000000000, -1.000000000000000000, 0.000000000000000000 ) ) ;
#16004=DIRECTION ( 'NONE',  ( -0.000000000000000000, -1.000000000000000000, 0.000000000000000000 ) ) ;
#16008=FACE_OUTER_BOUND ( 'NONE', #15976, .T. ) ;
#16028=ORIENTED_EDGE ( 'NONE', *, *, #10546, .T. ) ;
#16029=CARTESIAN_POINT ( 'NONE',  ( -12.90214402394279603, 13.86454579224779948, 47.04930799450052348 ) ) ;
#16039=ADVANCED_FACE ( 'NONE', ( #7667 ), #27959, .F. ) ;
#16040=EDGE_CURVE ( 'NONE', #12208, #20299, #24273, .T. ) ;
#16058=CARTESIAN_POINT ( 'NONE',  ( -6.902144023942790696, -5.098646251524523443, 47.04930799450052348 ) ) ;
#16070=DIRECTION ( 'NONE',  ( -1.000000000000000000, 0.000000000000000000, 0.000000000000000000 ) ) ;
#16071=TOROIDAL_SURFACE ( 'NONE', #5068, 46.69263079098917046, 1.200000000000001954 ) ;
#16082=DIRECTION ( 'NONE',  ( -0.000000000000000000, -1.000000000000000000, 0.000000000000000000 ) ) ;
#16084=DIRECTION ( 'NONE',  ( -1.000000000000000000, 0.000000000000000000, 0.000000000000000000 ) ) ;
#16085=AXIS2_PLACEMENT_3D ( 'NONE', #9984, #15660, #10599 ) ;
#16086=EDGE_LOOP ( 'NONE', ( #16488, #25924, #31141, #24271 ) ) ;
#16105=DIRECTION ( 'NONE',  ( -0.000000000000000000, -1.000000000000000000, 0.000000000000000000 ) ) ;
#16118=ORIENTED_EDGE ( 'NONE', *, *, #1705, .F. ) ;
#16133=AXIS2_PLACEMENT_3D ( 'NONE', #26476, #8440, #28618 ) ;
#16135=ORIENTED_EDGE ( 'NONE', *, *, #28030, .T. ) ;
#16136=DIRECTION ( 'NONE',  ( -0.000000000000000000, -1.000000000000000000, 0.000000000000000000 ) ) ;
#16140=ORIENTED_EDGE ( 'NONE', *, *, #5496, .T. ) ;
#16147=ORIENTED_EDGE ( 'NONE', *, *, #27476, .T. ) ;
#16167=EDGE_CURVE ( 'NONE', #5653, #490, #30591, .T. ) ;
#16194=ORIENTED_EDGE ( 'NONE', *, *, #13754, .T. ) ;
#16219=DIRECTION ( 'NONE',  ( -0.000000000000000000, -1.000000000000000000, 0.000000000000000000 ) ) ;
#16220=ADVANCED_FACE ( 'NONE', ( #29247 ), #24747, .F. ) ;
#16226=ORIENTED_EDGE ( 'NONE', *, *, #2929, .F. ) ;
#16235=TOROIDAL_SURFACE ( 'NONE', #7868, 46.67448298906162307, 0.7000000000000006217 ) ;
#16256=DIRECTION ( 'NONE',  ( -0.000000000000000000, -1.000000000000000000, 0.000000000000000000 ) ) ;
#16271=AXIS2_PLACEMENT_3D ( 'NONE', #6501, #4360, #31454 ) ;
#16272=DIRECTION ( 'NONE',  ( -1.000000000000000000, 0.000000000000000000, 0.000000000000000000 ) ) ;
#16280=AXIS2_PLACEMENT_3D ( 'NONE', #23765, #6212, #13608 ) ;
#16293=VERTEX_POINT ( 'NONE', #9068 ) ;
#16305=ORIENTED_EDGE ( 'NONE', *, *, #28401, .T. ) ;
#16306=CARTESIAN_POINT ( 'NONE',  ( 60.59785597605719687, 13.86454579224779948, 47.04930799450051637 ) ) ;
#16308=CARTESIAN_POINT ( 'NONE',  ( 21.09785597605720753, 14.99513937955032716, 47.04930799450052348 ) ) ;
#16324=AXIS2_PLACEMENT_3D ( 'NONE', #19733, #19574, #15150 ) ;
#16327=ORIENTED_EDGE ( 'NONE', *, *, #9005, .F. ) ;
#16333=DIRECTION ( 'NONE',  ( -0.000000000000000000, -1.000000000000000000, 0.000000000000000000 ) ) ;
#16346=ADVANCED_FACE ( 'NONE', ( #7432 ), #20617, .F. ) ;
#16352=ORIENTED_EDGE ( 'NONE', *, *, #26065, .T. ) ;
#16361=DIRECTION ( 'NONE',  ( -1.000000000000000000, 0.000000000000000000, 0.000000000000000000 ) ) ;
#16367=DIRECTION ( 'NONE',  ( -0.000000000000000000, -1.000000000000000000, 0.000000000000000000 ) ) ;
#16370=FACE_OUTER_BOUND ( 'NONE', #18328, .T. ) ;
#16382=DIRECTION ( 'NONE',  ( -0.000000000000000000, -1.000000000000000000, 0.000000000000000000 ) ) ;
#16388=DIRECTION ( 'NONE',  ( -1.000000000000000000, 0.000000000000000000, 0.000000000000000000 ) ) ;
#16393=AXIS2_PLACEMENT_3D ( 'NONE', #29515, #14412, #6536 ) ;
#16396=AXIS2_PLACEMENT_3D ( 'NONE', #26720, #16537, #14095 ) ;
#16402=EDGE_CURVE ( 'NONE', #19851, #12159, #15454, .T. ) ;
#16422=FACE_OUTER_BOUND ( 'NONE', #15304, .T. ) ;
#16438=EDGE_CURVE ( 'NONE', #7765, #294, #28964, .T. ) ;
#16442=EDGE_LOOP ( 'NONE', ( #14047, #22519, #10597, #6133 ) ) ;
#16446=DIRECTION ( 'NONE',  ( 1.000000000000000000, 0.000000000000000000, 0.000000000000000000 ) ) ;
#16449=CARTESIAN_POINT ( 'NONE',  ( 21.09785597605720753, 14.86454579224779948, 47.04930799450052348 ) ) ;
#16475=ADVANCED_FACE ( 'NONE', ( #13165 ), #21099, .F. ) ;
#16477=VERTEX_POINT ( 'NONE', #23162 ) ;
#16488=ORIENTED_EDGE ( 'NONE', *, *, #8967, .F. ) ;
#16491=AXIS2_PLACEMENT_3D ( 'NONE', #11478, #29042, #6561 ) ;
#16530=ORIENTED_EDGE ( 'NONE', *, *, #24008, .F. ) ;
#16532=CARTESIAN_POINT ( 'NONE',  ( 34.29963999142011488, 17.16467605102632632, 47.04930799450052348 ) ) ;
#16537=DIRECTION ( 'NONE',  ( -0.000000000000000000, -1.000000000000000000, 0.000000000000000000 ) ) ;
#16557=CARTESIAN_POINT ( 'NONE',  ( 21.09785597605720753, 13.86454579224779948, 47.04930799450052348 ) ) ;
#16583=DIRECTION ( 'NONE',  ( -1.000000000000000000, 0.000000000000000000, 0.000000000000000000 ) ) ;
#16621=AXIS2_PLACEMENT_3D ( 'NONE', #14832, #12372, #22359 ) ;
#16629=ORIENTED_EDGE ( 'NONE', *, *, #29770, .F. ) ;
#16634=CARTESIAN_POINT ( 'NONE',  ( 21.09785597605720753, -5.098646251524523443, 47.04930799450052348 ) ) ;
#16638=CARTESIAN_POINT ( 'NONE',  ( 21.09785597605720753, 14.86454579224779948, 47.04930799450052348 ) ) ;
#16647=DIRECTION ( 'NONE',  ( -0.000000000000000000, -1.000000000000000000, 0.000000000000000000 ) ) ;
#16666=VECTOR ( 'NONE', #22089, 1000.000000000000114 ) ;
#16680=DIRECTION ( 'NONE',  ( -0.000000000000000000, -1.000000000000000000, 0.000000000000000000 ) ) ;
#16687=CIRCLE ( 'NONE', #2556, 46.03812797983318461 ) ;
#16688=DIRECTION ( 'NONE',  ( -1.000000000000000000, 0.000000000000000000, 0.000000000000000000 ) ) ;
#16690=CARTESIAN_POINT ( 'NONE',  ( -3.902144023942795581, 14.86454579224779948, 47.04930799450052348 ) ) ;
#16697=DIRECTION ( 'NONE',  ( -0.000000000000000000, -1.000000000000000000, 0.000000000000000000 ) ) ;
#16716=CYLINDRICAL_SURFACE ( 'NONE', #2010, 25.50000000000000355 ) ;
#16729=CARTESIAN_POINT ( 'NONE',  ( 52.59785597605720397, 14.86454579224779948, 47.04930799450051637 ) ) ;
#16737=EDGE_CURVE ( 'NONE', #17055, #11782, #12482, .T. ) ;
#16749=AXIS2_PLACEMENT_3D ( 'NONE', #21637, #14272, #9013 ) ;
#16792=CARTESIAN_POINT ( 'NONE',  ( 21.09785597605720753, 17.36474115922713324, 47.04930799450052348 ) ) ;
#16804=CARTESIAN_POINT ( 'NONE',  ( 56.59785597605721108, 14.86454579224779948, 47.04930799450051637 ) ) ;
#16810=CYLINDRICAL_SURFACE ( 'NONE', #28081, 13.50178401536290806 ) ;
#16815=VERTEX_POINT ( 'NONE', #20980 ) ;
#16816=CARTESIAN_POINT ( 'NONE',  ( 21.09785597605720753, 14.86454579224779948, 47.04930799450052348 ) ) ;
#16817=DIRECTION ( 'NONE',  ( -1.000000000000000000, 0.000000000000000000, 0.000000000000000000 ) ) ;
#16819=DIRECTION ( 'NONE',  ( -1.000000000000000000, 0.000000000000000000, 0.000000000000000000 ) ) ;
#16828=ADVANCED_FACE ( 'NONE', ( #31008 ), #13786, .F. ) ;
#16837=EDGE_CURVE ( 'NONE', #18936, #15519, #29501, .T. ) ;
#16883=ORIENTED_EDGE ( 'NONE', *, *, #11399, .T. ) ;
#16906=CARTESIAN_POINT ( 'NONE',  ( 54.59785597605721108, -5.098646251524523443, 47.04930799450051637 ) ) ;
#16920=DIRECTION ( 'NONE',  ( 0.000000000000000000, 0.000000000000000000, 1.000000000000000000 ) ) ;
#16933=CIRCLE ( 'NONE', #25847, 13.30165371409683850 ) ;
#16967=FACE_OUTER_BOUND ( 'NONE', #26691, .T. ) ;
#16986=ORIENTED_EDGE ( 'NONE', *, *, #12545, .T. ) ;
#16987=EDGE_CURVE ( 'NONE', #10568, #17364, #31105, .T. ) ;
#17004=DIRECTION ( 'NONE',  ( 0.000000000000000000, 0.000000000000000000, 1.000000000000000000 ) ) ;
#17055=VERTEX_POINT ( 'NONE', #16690 ) ;
#17062=ADVANCED_FACE ( 'NONE', ( #31325 ), #20596, .T. ) ;
#17079=DIRECTION ( 'NONE',  ( -1.000000000000000000, 0.000000000000000000, 0.000000000000000000 ) ) ;
#17081=AXIS2_PLACEMENT_3D ( 'NONE', #5998, #16004, #26009 ) ;
#17095=LINE ( 'NONE', #14492, #11601 ) ;
#17098=DIRECTION ( 'NONE',  ( -1.000000000000000000, 0.000000000000000000, 0.000000000000000000 ) ) ;
#17125=DIRECTION ( 'NONE',  ( -1.000000000000000000, 0.000000000000000000, 0.000000000000000000 ) ) ;
#17136=CIRCLE ( 'NONE', #28674, 46.53489018157424084 ) ;
#17154=EDGE_CURVE ( 'NONE', #9965, #1158, #25860, .T. ) ;
#17158=AXIS2_PLACEMENT_3D ( 'NONE', #20257, #22885, #30452 ) ;
#17200=AXIS2_PLACEMENT_3D ( 'NONE', #27797, #25337, #20240 ) ;
#17203=ADVANCED_FACE ( 'NONE', ( #9813 ), #8054, .F. ) ;
#17207=CARTESIAN_POINT ( 'NONE',  ( 21.09785597605720753, 14.86454579224779948, 47.04930799450052348 ) ) ;
#17227=DIRECTION ( 'NONE',  ( -1.000000000000000000, 0.000000000000000000, 0.000000000000000000 ) ) ;
#17230=VERTEX_POINT ( 'NONE', #2749 ) ;
#17235=DIRECTION ( 'NONE',  ( -0.000000000000000000, -1.000000000000000000, 0.000000000000000000 ) ) ;
#17247=CARTESIAN_POINT ( 'NONE',  ( 21.09785597605720753, 14.36454579224779948, 47.04930799450052348 ) ) ;
#17255=DIRECTION ( 'NONE',  ( -0.000000000000000000, -1.000000000000000000, 0.000000000000000000 ) ) ;
#17258=CARTESIAN_POINT ( 'NONE',  ( 34.59963999142011204, -5.098646251524523443, 47.04930799450052348 ) ) ;
#17268=CIRCLE ( 'NONE', #28800, 13.31487396812510937 ) ;
#17273=DIRECTION ( 'NONE',  ( -0.000000000000000000, -1.000000000000000000, 0.000000000000000000 ) ) ;
#17281=CARTESIAN_POINT ( 'NONE',  ( 7.096071960694297687, 16.03967147762300982, 47.04930799450052348 ) ) ;
#17289=AXIS2_PLACEMENT_3D ( 'NONE', #5923, #20686, #25772 ) ;
#17290=EDGE_CURVE ( 'NONE', #23918, #24672, #17986, .T. ) ;
#17292=CIRCLE ( 'NONE', #30414, 13.31487396812510937 ) ;
#17296=VECTOR ( 'NONE', #20388, 1000.000000000000000 ) ;
#17304=ORIENTED_EDGE ( 'NONE', *, *, #161, .T. ) ;
#17364=VERTEX_POINT ( 'NONE', #11115 ) ;
#17392=FACE_OUTER_BOUND ( 'NONE', #3857, .T. ) ;
#17404=CARTESIAN_POINT ( 'NONE',  ( 21.09785597605720753, 14.86454579224779948, 47.04930799450052348 ) ) ;
#17407=EDGE_CURVE ( 'NONE', #18982, #5510, #4196, .T. ) ;
#17420=EDGE_CURVE ( 'NONE', #13945, #2441, #7000, .T. ) ;
#17433=DIRECTION ( 'NONE',  ( -1.000000000000000000, 0.000000000000000000, 0.000000000000000000 ) ) ;
#17443=ORIENTED_EDGE ( 'NONE', *, *, #2605, .T. ) ;
#17466=EDGE_LOOP ( 'NONE', ( #19149, #13877, #22768, #29439 ) ) ;
#17478=AXIS2_PLACEMENT_3D ( 'NONE', #31290, #24048, #11747 ) ;
#17490=VECTOR ( 'NONE', #5985, 1000.000000000000000 ) ;
#17504=CIRCLE ( 'NONE', #23752, 1.499999999999994449 ) ;
#17507=CARTESIAN_POINT ( 'NONE',  ( 21.09785597605720753, 14.86454579224779948, 47.04930799450052348 ) ) ;
#17526=ORIENTED_EDGE ( 'NONE', *, *, #17533, .F. ) ;
#17533=EDGE_CURVE ( 'NONE', #26331, #7154, #1225, .T. ) ;
#17541=CYLINDRICAL_SURFACE ( 'NONE', #25124, 27.49999999999999289 ) ;
#17549=CIRCLE ( 'NONE', #30147, 27.99999999999999645 ) ;
#17555=CARTESIAN_POINT ( 'NONE',  ( 21.09785597605720753, 14.86454579224779948, 47.04930799450052348 ) ) ;
#17556=DIRECTION ( 'NONE',  ( -0.000000000000000000, -1.000000000000000000, 0.000000000000000000 ) ) ;
#17569=CIRCLE ( 'NONE', #6558, 1.499999999999997780 ) ;
#17581=FACE_OUTER_BOUND ( 'NONE', #32032, .T. ) ;
#17608=CARTESIAN_POINT ( 'NONE',  ( 21.09785597605720753, 14.81645899701909563, 47.04930799450052348 ) ) ;
#17611=VECTOR ( 'NONE', #13957, 1000.000000000000000 ) ;
#17616=AXIS2_PLACEMENT_3D ( 'NONE', #2142, #10024, #27416 ) ;
#17631=ADVANCED_FACE ( 'NONE', ( #27961 ), #5479, .F. ) ;
#17633=DIRECTION ( 'NONE',  ( -1.000000000000000000, 0.000000000000000000, 0.000000000000000000 ) ) ;
#17637=FACE_OUTER_BOUND ( 'NONE', #21971, .T. ) ;
#17639=DIRECTION ( 'NONE',  ( -1.000000000000000000, 0.000000000000000000, 0.000000000000000000 ) ) ;
#17649=EDGE_CURVE ( 'NONE', #10403, #25889, #11050, .T. ) ;
#17650=CIRCLE ( 'NONE', #5073, 28.00000000000000000 ) ;
#17663=VERTEX_POINT ( 'NONE', #23021 ) ;
#17664=CARTESIAN_POINT ( 'NONE',  ( 5.864109918520784781, 14.46497581658974063, 47.04930799450052348 ) ) ;
#17667=CARTESIAN_POINT ( 'NONE',  ( -25.30045392157957096, 13.78442380691147839, 47.04930799450052348 ) ) ;
#17675=EDGE_CURVE ( 'NONE', #22149, #10005, #18613, .T. ) ;
#17677=CARTESIAN_POINT ( 'NONE',  ( 21.09785597605720753, 16.03967147762300982, 47.04930799450052348 ) ) ;
#17680=LINE ( 'NONE', #27699, #30303 ) ;
#17700=ORIENTED_EDGE ( 'NONE', *, *, #30428, .F. ) ;
#17701=AXIS2_PLACEMENT_3D ( 'NONE', #26565, #29035, #6386 ) ;
#17705=EDGE_CURVE ( 'NONE', #17230, #12393, #12339, .T. ) ;
#17709=ADVANCED_FACE ( 'NONE', ( #22057 ), #24522, .F. ) ;
#17716=DIRECTION ( 'NONE',  ( -0.000000000000000000, -1.000000000000000000, 0.000000000000000000 ) ) ;
#17719=CARTESIAN_POINT ( 'NONE',  ( 21.09785597605720753, 13.86454579224779948, 47.04930799450052348 ) ) ;
#17723=DIRECTION ( 'NONE',  ( -1.000000000000000000, 0.000000000000000000, 0.000000000000000000 ) ) ;
#17725=CARTESIAN_POINT ( 'NONE',  ( 46.09785597605720397, 14.86454579224779948, 47.04930799450052348 ) ) ;
#17729=ORIENTED_EDGE ( 'NONE', *, *, #4782, .T. ) ;
#17730=TOROIDAL_SURFACE ( 'NONE', #16133, 38.50000000000000000, 1.499999999999997780 ) ;
#17776=ADVANCED_FACE ( 'NONE', ( #16967 ), #16810, .T. ) ;
#17816=AXIS2_PLACEMENT_3D ( 'NONE', #26485, #21710, #11232 ) ;
#17818=EDGE_CURVE ( 'NONE', #15519, #29185, #3941, .T. ) ;
#17832=CARTESIAN_POINT ( 'NONE',  ( 21.09785597605720753, 15.23758267881771111, 47.04930799450052348 ) ) ;
#17852=ORIENTED_EDGE ( 'NONE', *, *, #27579, .F. ) ;
#17866=AXIS2_PLACEMENT_3D ( 'NONE', #6012, #3374, #13408 ) ;
#17868=CIRCLE ( 'NONE', #1095, 0.9999999999999974465 ) ;
#17870=FACE_OUTER_BOUND ( 'NONE', #10377, .T. ) ;
#17883=DIRECTION ( 'NONE',  ( -1.000000000000000000, 0.000000000000000000, 0.000000000000000000 ) ) ;
#17892=ORIENTED_EDGE ( 'NONE', *, *, #26249, .F. ) ;
#17915=DIRECTION ( 'NONE',  ( -1.000000000000000000, 0.000000000000000000, 0.000000000000000000 ) ) ;
#17919=VERTEX_POINT ( 'NONE', #5330 ) ;
#17931=VERTEX_POINT ( 'NONE', #24857 ) ;
#17937=VECTOR ( 'NONE', #32062, 1000.000000000000000 ) ;
#17964=EDGE_LOOP ( 'NONE', ( #6876, #13827, #7438, #4041 ) ) ;
#17980=EDGE_CURVE ( 'NONE', #17663, #12804, #10741, .T. ) ;
#17986=CIRCLE ( 'NONE', #29554, 13.00178401536290806 ) ;
#17997=EDGE_LOOP ( 'NONE', ( #7196, #26345, #22441, #5914 ) ) ;
#18036=DIRECTION ( 'NONE',  ( -1.000000000000000000, 0.000000000000000000, 0.000000000000000000 ) ) ;
#18038=ORIENTED_EDGE ( 'NONE', *, *, #4536, .F. ) ;
#18039=CARTESIAN_POINT ( 'NONE',  ( 34.59963999142011204, 17.16474120167318063, 47.04930799450052348 ) ) ;
#18040=EDGE_CURVE ( 'NONE', #15519, #7154, #8101, .T. ) ;
#18056=VERTEX_POINT ( 'NONE', #13683 ) ;
#18057=AXIS2_PLACEMENT_3D ( 'NONE', #27029, #4542, #2079 ) ;
#18061=FACE_OUTER_BOUND ( 'NONE', #1191, .T. ) ;
#18063=ORIENTED_EDGE ( 'NONE', *, *, #201, .T. ) ;
#18064=DIRECTION ( 'NONE',  ( 1.000000000000000000, 0.000000000000000000, 0.000000000000000000 ) ) ;
#18067=CARTESIAN_POINT ( 'NONE',  ( 21.09785597605720753, 13.86454579224779948, 47.04930799450052348 ) ) ;
#18069=CARTESIAN_POINT ( 'NONE',  ( 21.09785597605720753, 14.86454579224779948, 47.04930799450052348 ) ) ;
#18072=CARTESIAN_POINT ( 'NONE',  ( 52.09785597605720397, 13.86454579224779948, 47.04930799450051637 ) ) ;
#18075=SHAPE_REPRESENTATION_RELATIONSHIP ( 'NONE' , 'NONE' ,  #11371, #4182 ) ;
#18077=VERTEX_POINT ( 'NONE', #3333 ) ;
#18080=EDGE_CURVE ( 'NONE', #21342, #30851, #3816, .T. ) ;
#18087=ORIENTED_EDGE ( 'NONE', *, *, #16987, .T. ) ;
#18092=CIRCLE ( 'NONE', #12337, 0.9999999999999974465 ) ;
#18095=AXIS2_PLACEMENT_3D ( 'NONE', #1719, #11735, #21731 ) ;
#18100=AXIS2_PLACEMENT_3D ( 'NONE', #11442, #21440, #8983 ) ;
#18105=DIRECTION ( 'NONE',  ( -1.000000000000000000, 0.000000000000000000, 0.000000000000000000 ) ) ;
#18139=ORIENTED_EDGE ( 'NONE', *, *, #17649, .T. ) ;
#18175=DIRECTION ( 'NONE',  ( -1.000000000000000000, 0.000000000000000000, 0.000000000000000000 ) ) ;
#18196=DIRECTION ( 'NONE',  ( -0.000000000000000000, -1.000000000000000000, 0.000000000000000000 ) ) ;
#18199=CIRCLE ( 'NONE', #20831, 40.00000000000000000 ) ;
#18228=ORIENTED_EDGE ( 'NONE', *, *, #12660, .F. ) ;
#18233=VERTEX_POINT ( 'NONE', #15133 ) ;
#18247=EDGE_LOOP ( 'NONE', ( #12965, #18063, #20271, #19964 ) ) ;
#18256=TOROIDAL_SURFACE ( 'NONE', #13038, 54.10000000000000142, 0.1999999999999993727 ) ;
#18269=FACE_OUTER_BOUND ( 'NONE', #12244, .T. ) ;
#18271=DIRECTION ( 'NONE',  ( -1.000000000000000000, 0.000000000000000000, 0.000000000000000000 ) ) ;
#18287=AXIS2_PLACEMENT_3D ( 'NONE', #17207, #27225, #13961 ) ;
#18295=DIRECTION ( 'NONE',  ( -1.000000000000000000, 0.000000000000000000, 0.000000000000000000 ) ) ;
#18300=ORIENTED_EDGE ( 'NONE', *, *, #14028, .T. ) ;
#18313=CIRCLE ( 'NONE', #28792, 19.50000000000000000 ) ;
#18318=ORIENTED_EDGE ( 'NONE', *, *, #22746, .T. ) ;
#18328=EDGE_LOOP ( 'NONE', ( #26944, #19399, #10650, #30819 ) ) ;
#18334=ADVANCED_FACE ( 'NONE', ( #19717 ), #2491, .F. ) ;
#18349=ORIENTED_EDGE ( 'NONE', *, *, #29393, .T. ) ;
#18363=DIRECTION ( 'NONE',  ( -0.000000000000000000, -1.000000000000000000, 0.000000000000000000 ) ) ;
#18365=CIRCLE ( 'NONE', #25716, 39.50000000000000000 ) ;
#18371=ORIENTED_EDGE ( 'NONE', *, *, #27675, .T. ) ;
#18374=EDGE_CURVE ( 'NONE', #28560, #22190, #20151, .T. ) ;
#18398=AXIS2_PLACEMENT_3D ( 'NONE', #1363, #28778, #6620 ) ;
#18412=CIRCLE ( 'NONE', #5853, 13.50178401536290984 ) ;
#18440=DIRECTION ( 'NONE',  ( -1.000000000000000000, 0.000000000000000000, 0.000000000000000000 ) ) ;
#18462=DIRECTION ( 'NONE',  ( -1.000000000000000000, 0.000000000000000000, 0.000000000000000000 ) ) ;
#18503=CIRCLE ( 'NONE', #16396, 43.50000000000000000 ) ;
#18512=DIRECTION ( 'NONE',  ( 1.000000000000000000, 0.000000000000000000, 0.000000000000000000 ) ) ;
#18553=ADVANCED_FACE ( 'NONE', ( #29331 ), #13373, .T. ) ;
#18559=ORIENTED_EDGE ( 'NONE', *, *, #5225, .T. ) ;
#18575=CARTESIAN_POINT ( 'NONE',  ( 21.09785597605720753, 15.70210863493540288, 47.04930799450052348 ) ) ;
#18576=EDGE_CURVE ( 'NONE', #18781, #13490, #17549, .T. ) ;
#18592=CARTESIAN_POINT ( 'NONE',  ( 0.5978559760572086379, 13.86454579224779948, 47.04930799450052348 ) ) ;
#18613=CIRCLE ( 'NONE', #4481, 0.2551199516247909527 ) ;
#18617=EDGE_CURVE ( 'NONE', #16477, #10620, #15441, .T. ) ;
#18628=ORIENTED_EDGE ( 'NONE', *, *, #13754, .F. ) ;
#18643=DIRECTION ( 'NONE',  ( -0.000000000000000000, -1.000000000000000000, 0.000000000000000000 ) ) ;
#18652=VERTEX_POINT ( 'NONE', #17664 ) ;
#18666=ORIENTED_EDGE ( 'NONE', *, *, #16402, .F. ) ;
#18668=AXIS2_PLACEMENT_3D ( 'NONE', #3688, #8298, #18295 ) ;
#18682=ORIENTED_EDGE ( 'NONE', *, *, #23970, .T. ) ;
#18700=ORIENTED_EDGE ( 'NONE', *, *, #21978, .T. ) ;
#18708=ORIENTED_EDGE ( 'NONE', *, *, #29128, .F. ) ;
#18747=CIRCLE ( 'NONE', #3581, 54.30000000000000426 ) ;
#18750=DIRECTION ( 'NONE',  ( -1.000000000000000000, 0.000000000000000000, 0.000000000000000000 ) ) ;
#18756=CARTESIAN_POINT ( 'NONE',  ( 21.09785597605720753, 13.86454579224779948, 47.04930799450052348 ) ) ;
#18765=CIRCLE ( 'NONE', #4637, 1.500000000000001332 ) ;
#18778=FACE_OUTER_BOUND ( 'NONE', #18948, .T. ) ;
#18781=VERTEX_POINT ( 'NONE', #1079 ) ;
#18785=ORIENTED_EDGE ( 'NONE', *, *, #30440, .F. ) ;
#18800=ORIENTED_EDGE ( 'NONE', *, *, #16167, .T. ) ;
#18804=VERTEX_POINT ( 'NONE', #8782 ) ;
#18822=DIRECTION ( 'NONE',  ( -0.000000000000000000, -1.000000000000000000, 0.000000000000000000 ) ) ;
#18838=ORIENTED_EDGE ( 'NONE', *, *, #5753, .T. ) ;
#18839=FACE_OUTER_BOUND ( 'NONE', #7501, .T. ) ;
#18846=EDGE_CURVE ( 'NONE', #2312, #18936, #20195, .T. ) ;
#18860=CARTESIAN_POINT ( 'NONE',  ( -25.18206523986666312, 14.81645899701909563, 47.04930799450052348 ) ) ;
#18868=EDGE_CURVE ( 'NONE', #10602, #9753, #18092, .T. ) ;
#18875=DIRECTION ( 'NONE',  ( -0.000000000000000000, -1.000000000000000000, 0.000000000000000000 ) ) ;
#18886=CARTESIAN_POINT ( 'NONE',  ( 21.09785597605720753, 13.86454579224779948, 47.04930799450052348 ) ) ;
#18899=CARTESIAN_POINT ( 'NONE',  ( 48.59785597605720397, 14.86454579224779948, 47.04930799450052348 ) ) ;
#18900=VECTOR ( 'NONE', #31124, 1000.000000000000000 ) ;
#18901=LINE ( 'NONE', #1505, #8389 ) ;
#18917=CARTESIAN_POINT ( 'NONE',  ( 21.09785597605720753, 14.05098971466613023, 47.04930799450052348 ) ) ;
#18925=AXIS2_PLACEMENT_3D ( 'NONE', #8961, #23896, #31933 ) ;
#18936=VERTEX_POINT ( 'NONE', #26510 ) ;
#18945=CARTESIAN_POINT ( 'NONE',  ( 21.09785597605720753, 14.46497581658974063, 47.04930799450052348 ) ) ;
#18948=EDGE_LOOP ( 'NONE', ( #7865, #30694, #16147, #23655 ) ) ;
#18949=CARTESIAN_POINT ( 'NONE',  ( 67.18867716679213231, 14.05098971466613023, 47.04930799450051637 ) ) ;
#18953=VERTEX_POINT ( 'NONE', #21898 ) ;
#18954=FACE_OUTER_BOUND ( 'NONE', #2890, .T. ) ;
#18958=AXIS2_PLACEMENT_3D ( 'NONE', #9933, #19446, #31768 ) ;
#18962=AXIS2_PLACEMENT_3D ( 'NONE', #26017, #11531, #22014 ) ;
#18980=EDGE_CURVE ( 'NONE', #10403, #13364, #28054, .T. ) ;
#18982=VERTEX_POINT ( 'NONE', #9444 ) ;
#18998=DIRECTION ( 'NONE',  ( -1.000000000000000000, 0.000000000000000000, 0.000000000000000000 ) ) ;
#19010=CIRCLE ( 'NONE', #5432, 37.50000000000000711 ) ;
#19018=ORIENTED_EDGE ( 'NONE', *, *, #21024, .F. ) ;
#19020=DIRECTION ( 'NONE',  ( -1.000000000000000000, 0.000000000000000000, 0.000000000000000000 ) ) ;
#19031=ORIENTED_EDGE ( 'NONE', *, *, #26381, .F. ) ;
#19056=DIRECTION ( 'NONE',  ( 1.000000000000000000, 0.000000000000000000, 0.000000000000000000 ) ) ;
#19058=CARTESIAN_POINT ( 'NONE',  ( 75.39785597605721534, 14.66454579224779842, 47.04930799450051637 ) ) ;
#19072=CIRCLE ( 'NONE', #15952, 2.000000000000001776 ) ;
#19077=ORIENTED_EDGE ( 'NONE', *, *, #21024, .T. ) ;
#19079=TOROIDAL_SURFACE ( 'NONE', #27490, 29.50000000000000355, 2.000000000000001776 ) ;
#19083=DIRECTION ( 'NONE',  ( -1.000000000000000000, 0.000000000000000000, 0.000000000000000000 ) ) ;
#19089=ADVANCED_FACE ( 'NONE', ( #6128 ), #28079, .T. ) ;
#19107=LINE ( 'NONE', #1231, #13202 ) ;
#19129=VERTEX_POINT ( 'NONE', #1192 ) ;
#19146=ORIENTED_EDGE ( 'NONE', *, *, #7356, .F. ) ;
#19149=ORIENTED_EDGE ( 'NONE', *, *, #7275, .F. ) ;
#19168=VERTEX_POINT ( 'NONE', #3825 ) ;
#19212=DIRECTION ( 'NONE',  ( -1.000000000000000000, 0.000000000000000000, 0.000000000000000000 ) ) ;
#19213=VECTOR ( 'NONE', #6622, 1000.000000000000000 ) ;
#19230=CARTESIAN_POINT ( 'NONE',  ( 40.09785597605721108, -5.098646251524523443, 47.04930799450052348 ) ) ;
#19237=CYLINDRICAL_SURFACE ( 'NONE', #9097, 27.99999999999999645 ) ;
#19264=FACE_OUTER_BOUND ( 'NONE', #29777, .T. ) ;
#19269=DIRECTION ( 'NONE',  ( 1.000000000000000000, 0.000000000000000000, 0.000000000000000000 ) ) ;
#19272=CARTESIAN_POINT ( 'NONE',  ( 21.09785597605720753, 17.16467605102632632, 47.04930799450052348 ) ) ;
#19296=AXIS2_PLACEMENT_3D ( 'NONE', #18575, #30599, #15640 ) ;
#19315=CARTESIAN_POINT ( 'NONE',  ( 47.59785597605720397, 13.86454579224779948, 47.04930799450052348 ) ) ;
#19321=DIRECTION ( 'NONE',  ( -0.000000000000000000, -1.000000000000000000, 0.000000000000000000 ) ) ;
#19326=CIRCLE ( 'NONE', #14114, 45.49665035954053138 ) ;
#19336=EDGE_CURVE ( 'NONE', #21342, #23289, #12912, .T. ) ;
#19343=CARTESIAN_POINT ( 'NONE',  ( -9.902144023942796025, 14.86454579224779948, 47.04930799450052348 ) ) ;
#19348=DIRECTION ( 'NONE',  ( -0.000000000000000000, -1.000000000000000000, 0.000000000000000000 ) ) ;
#19353=ORIENTED_EDGE ( 'NONE', *, *, #26381, .T. ) ;
#19361=CARTESIAN_POINT ( 'NONE',  ( 21.09785597605720753, 17.16467605102632632, 47.04930799450052348 ) ) ;
#19365=ORIENTED_EDGE ( 'NONE', *, *, #9342, .T. ) ;
#19371=CIRCLE ( 'NONE', #5750, 46.09082119073493544 ) ;
#19391=VECTOR ( 'NONE', #23790, 1000.000000000000000 ) ;
#19393=CARTESIAN_POINT ( 'NONE',  ( -16.40214402394279958, 13.86454579224779948, 47.04930799450052348 ) ) ;
#19399=ORIENTED_EDGE ( 'NONE', *, *, #6520, .T. ) ;
#19401=ADVANCED_FACE ( 'NONE', ( #30245 ), #5550, .T. ) ;
#19412=ORIENTED_EDGE ( 'NONE', *, *, #4996, .F. ) ;
#19418=DIRECTION ( 'NONE',  ( 1.000000000000000000, 0.000000000000000000, 0.000000000000000000 ) ) ;
#19426=VECTOR ( 'NONE', #28621, 1000.000000000000000 ) ;
#19446=DIRECTION ( 'NONE',  ( -0.000000000000000000, -1.000000000000000000, 0.000000000000000000 ) ) ;
#19448=ADVANCED_FACE ( 'NONE', ( #23492 ), #23003, .T. ) ;
#19464=CIRCLE ( 'NONE', #31019, 1.500000000000001332 ) ;
#19471=CARTESIAN_POINT ( 'NONE',  ( -9.902144023942794249, 13.86454579224779948, 47.04930799450052348 ) ) ;
#19501=DIRECTION ( 'NONE',  ( -1.000000000000000000, 0.000000000000000000, 0.000000000000000000 ) ) ;
#19509=AXIS2_PLACEMENT_3D ( 'NONE', #20324, #24944, #15255 ) ;
#19511=CARTESIAN_POINT ( 'NONE',  ( 58.59785597605721108, 13.86454579224779948, 47.04930799450051637 ) ) ;
#19562=ADVANCED_FACE ( 'NONE', ( #24455 ), #23387, .T. ) ;
#19570=LINE ( 'NONE', #12201, #7740 ) ;
#19572=VERTEX_POINT ( 'NONE', #16729 ) ;
#19574=DIRECTION ( 'NONE',  ( -0.000000000000000000, -1.000000000000000000, 0.000000000000000000 ) ) ;
#19590=ADVANCED_FACE ( 'NONE', ( #9533 ), #1650, .T. ) ;
#19610=EDGE_LOOP ( 'NONE', ( #17892, #10134 ) ) ;
#19620=EDGE_CURVE ( 'NONE', #19851, #26545, #26527, .T. ) ;
#19623=AXIS2_PLACEMENT_3D ( 'NONE', #20516, #3105, #20345 ) ;
#19634=DIRECTION ( 'NONE',  ( -1.000000000000000000, 0.000000000000000000, 0.000000000000000000 ) ) ;
#19635=VERTEX_POINT ( 'NONE', #23805 ) ;
#19643=DIRECTION ( 'NONE',  ( -0.000000000000000000, -1.000000000000000000, 0.000000000000000000 ) ) ;
#19651=CARTESIAN_POINT ( 'NONE',  ( 2.097855976057206639, -5.098646251524523443, 47.04930799450052348 ) ) ;
#19679=CARTESIAN_POINT ( 'NONE',  ( 52.59785597605720397, 13.86454579224779948, 47.04930799450051637 ) ) ;
#19717=FACE_OUTER_BOUND ( 'NONE', #3882, .T. ) ;
#19723=CARTESIAN_POINT ( 'NONE',  ( -0.4021440239427923058, 14.86454579224779948, 47.04930799450052348 ) ) ;
#19729=AXIS2_PLACEMENT_3D ( 'NONE', #17247, #22336, #27263 ) ;
#19733=CARTESIAN_POINT ( 'NONE',  ( 21.09785597605720753, -5.098646251524523443, 47.04930799450052348 ) ) ;
#19735=EDGE_LOOP ( 'NONE', ( #2328, #7253, #20801, #26525 ) ) ;
#19737=DIRECTION ( 'NONE',  ( -0.000000000000000000, -1.000000000000000000, 0.000000000000000000 ) ) ;
#19738=CARTESIAN_POINT ( 'NONE',  ( -21.90214402394278892, -5.098646251524523443, 47.04930799450052348 ) ) ;
#19742=AXIS2_PLACEMENT_3D ( 'NONE', #8752, #16136, #18750 ) ;
#19747=EDGE_CURVE ( 'NONE', #10620, #16477, #22329, .T. ) ;
#19767=DIRECTION ( 'NONE',  ( -0.000000000000000000, -1.000000000000000000, 0.000000000000000000 ) ) ;
#19783=EDGE_CURVE ( 'NONE', #17931, #13599, #13440, .T. ) ;
#19784=EDGE_CURVE ( 'NONE', #2312, #30851, #8214, .T. ) ;
#19789=ORIENTED_EDGE ( 'NONE', *, *, #14720, .T. ) ;
#19809=DIRECTION ( 'NONE',  ( -0.000000000000000000, -1.000000000000000000, 0.000000000000000000 ) ) ;
#19829=ORIENTED_EDGE ( 'NONE', *, *, #12433, .T. ) ;
#19833=TOROIDAL_SURFACE ( 'NONE', #5703, 44.50000000000000000, 1.000000000000000000 ) ;
#19836=DIRECTION ( 'NONE',  ( -1.000000000000000000, 0.000000000000000000, 0.000000000000000000 ) ) ;
#19844=EDGE_CURVE ( 'NONE', #15722, #7100, #1377, .T. ) ;
#19851=VERTEX_POINT ( 'NONE', #18039 ) ;
#19861=VERTEX_POINT ( 'NONE', #15745 ) ;
#19866=ADVANCED_FACE ( 'NONE', ( #28549 ), #16071, .T. ) ;
#19869=CIRCLE ( 'NONE', #25131, 19.00000000000000000 ) ;
#19889=ORIENTED_EDGE ( 'NONE', *, *, #6818, .F. ) ;
#19924=EDGE_LOOP ( 'NONE', ( #17852, #8217, #30801, #28950 ) ) ;
#19935=FACE_OUTER_BOUND ( 'NONE', #29631, .T. ) ;
#19949=CIRCLE ( 'NONE', #8410, 0.9999999999999940048 ) ;
#19964=ORIENTED_EDGE ( 'NONE', *, *, #3361, .F. ) ;
#19974=DIRECTION ( 'NONE',  ( -1.000000000000000000, 0.000000000000000000, 0.000000000000000000 ) ) ;
#19991=EDGE_LOOP ( 'NONE', ( #27070, #6588, #29386, #2129 ) ) ;
#19998=EDGE_CURVE ( 'NONE', #31745, #12208, #12948, .T. ) ;
#20011=AXIS2_PLACEMENT_3D ( 'NONE', #22883, #393, #28301 ) ;
#20022=DIRECTION ( 'NONE',  ( 1.000000000000000000, 0.000000000000000000, 0.000000000000000000 ) ) ;
#20025=ORIENTED_EDGE ( 'NONE', *, *, #29698, .T. ) ;
#20027=AXIS2_PLACEMENT_3D ( 'NONE', #4516, #6980, #32098 ) ;
#20035=ORIENTED_EDGE ( 'NONE', *, *, #32281, .T. ) ;
#20038=EDGE_CURVE ( 'NONE', #10875, #22237, #32321, .T. ) ;
#20041=EDGE_CURVE ( 'NONE', #12393, #29883, #30750, .T. ) ;
#20056=CARTESIAN_POINT ( 'NONE',  ( 34.59963999142011204, 16.03967147762301693, 47.04930799450052348 ) ) ;
#20083=ORIENTED_EDGE ( 'NONE', *, *, #11399, .F. ) ;
#20090=ORIENTED_EDGE ( 'NONE', *, *, #24482, .T. ) ;
#20092=DIRECTION ( 'NONE',  ( -1.224646799147353207E-16, 0.000000000000000000, -1.000000000000000000 ) ) ;
#20105=AXIS2_PLACEMENT_3D ( 'NONE', #24654, #2173, #9234 ) ;
#20106=ORIENTED_EDGE ( 'NONE', *, *, #27476, .F. ) ;
#20125=CARTESIAN_POINT ( 'NONE',  ( 67.77233896511883415, 14.36454579224780126, 47.04930799450051637 ) ) ;
#20149=DIRECTION ( 'NONE',  ( -1.000000000000000000, 0.000000000000000000, 0.000000000000000000 ) ) ;
#20151=CIRCLE ( 'NONE', #783, 34.00000000000000000 ) ;
#20169=ORIENTED_EDGE ( 'NONE', *, *, #1891, .T. ) ;
#20184=DIRECTION ( 'NONE',  ( -0.000000000000000000, -1.000000000000000000, 0.000000000000000000 ) ) ;
#20189=CARTESIAN_POINT ( 'NONE',  ( 21.09785597605720753, -5.098646251524523443, 47.04930799450052348 ) ) ;
#20195=CIRCLE ( 'NONE', #5000, 1.200000000000003064 ) ;
#20199=ADVANCED_FACE ( 'NONE', ( #32469 ), #7525, .F. ) ;
#20206=ORIENTED_EDGE ( 'NONE', *, *, #22250, .F. ) ;
#20207=DIRECTION ( 'NONE',  ( -0.000000000000000000, -1.000000000000000000, 0.000000000000000000 ) ) ;
#20240=DIRECTION ( 'NONE',  ( -1.000000000000000000, 0.000000000000000000, 0.000000000000000000 ) ) ;
#20257=CARTESIAN_POINT ( 'NONE',  ( 21.09785597605720753, 13.78276522714992147, 47.04930799450052348 ) ) ;
#20258=DIRECTION ( 'NONE',  ( -1.000000000000000000, 0.000000000000000000, 0.000000000000000000 ) ) ;
#20259=ORIENTED_EDGE ( 'NONE', *, *, #17533, .T. ) ;
#20266=EDGE_CURVE ( 'NONE', #18233, #14305, #22907, .T. ) ;
#20271=ORIENTED_EDGE ( 'NONE', *, *, #12318, .T. ) ;
#20277=AXIS2_PLACEMENT_3D ( 'NONE', #15832, #6296, #13380 ) ;
#20283=EDGE_CURVE ( 'NONE', #7154, #26331, #17136, .T. ) ;
#20287=DIRECTION ( 'NONE',  ( -0.000000000000000000, -1.000000000000000000, 0.000000000000000000 ) ) ;
#20291=EDGE_CURVE ( 'NONE', #31745, #19168, #2993, .T. ) ;
#20292=CARTESIAN_POINT ( 'NONE',  ( 21.09785597605720753, -5.098646251524523443, 47.04930799450052348 ) ) ;
#20299=VERTEX_POINT ( 'NONE', #733 ) ;
#20308=TOROIDAL_SURFACE ( 'NONE', #29213, 46.67448298906162307, 0.7000000000000006217 ) ;
#20324=CARTESIAN_POINT ( 'NONE',  ( 21.09785597605720753, 14.86454579224779948, 47.04930799450052348 ) ) ;
#20333=CARTESIAN_POINT ( 'NONE',  ( -24.39879438348332386, 13.78276522714992147, 47.04930799450052348 ) ) ;
#20345=DIRECTION ( 'NONE',  ( -1.000000000000000000, 0.000000000000000000, 0.000000000000000000 ) ) ;
#20351=AXIS2_PLACEMENT_3D ( 'NONE', #25886, #775, #13424 ) ;
#20352=ORIENTED_EDGE ( 'NONE', *, *, #5461, .T. ) ;
#20357=ORIENTED_EDGE ( 'NONE', *, *, #18080, .F. ) ;
#20364=DIRECTION ( 'NONE',  ( -0.000000000000000000, -1.000000000000000000, 0.000000000000000000 ) ) ;
#20365=CYLINDRICAL_SURFACE ( 'NONE', #28379, 27.49999999999999289 ) ;
#20371=DIRECTION ( 'NONE',  ( -0.000000000000000000, -1.000000000000000000, 0.000000000000000000 ) ) ;
#20375=AXIS2_PLACEMENT_3D ( 'NONE', #20598, #8291, #742 ) ;
#20377=EDGE_CURVE ( 'NONE', #663, #25220, #14532, .T. ) ;
#20380=EDGE_CURVE ( 'NONE', #3892, #5653, #5602, .T. ) ;
#20388=DIRECTION ( 'NONE',  ( -0.000000000000000000, -1.000000000000000000, 0.000000000000000000 ) ) ;
#20397=AXIS2_PLACEMENT_3D ( 'NONE', #6648, #6972, #29292 ) ;
#20420=ORIENTED_EDGE ( 'NONE', *, *, #30472, .T. ) ;
#20465=AXIS2_PLACEMENT_3D ( 'NONE', #5252, #15261, #12812 ) ;
#20470=EDGE_CURVE ( 'NONE', #25220, #19861, #9246, .T. ) ;
#20479=ORIENTED_EDGE ( 'NONE', *, *, #23207, .T. ) ;
#20483=CIRCLE ( 'NONE', #16280, 31.50000000000000000 ) ;
#20488=ADVANCED_FACE ( 'NONE', ( #24668 ), #31838, .F. ) ;
#20499=ORIENTED_EDGE ( 'NONE', *, *, #29698, .F. ) ;
#20508=DIRECTION ( 'NONE',  ( -0.000000000000000000, -1.000000000000000000, 0.000000000000000000 ) ) ;
#20516=CARTESIAN_POINT ( 'NONE',  ( 21.09785597605720753, 14.86454579224779948, 47.04930799450052348 ) ) ;
#20518=AXIS2_PLACEMENT_3D ( 'NONE', #6492, #26347, #16817 ) ;
#20520=VERTEX_POINT ( 'NONE', #22520 ) ;
#20523=CARTESIAN_POINT ( 'NONE',  ( 21.09785597605720753, 17.16474120167318418, 47.04930799450052348 ) ) ;
#20531=AXIS2_PLACEMENT_3D ( 'NONE', #12706, #32229, #14993 ) ;
#20549=CARTESIAN_POINT ( 'NONE',  ( 21.09785597605720753, 13.66454579224780019, 47.04930799450052348 ) ) ;
#20552=ORIENTED_EDGE ( 'NONE', *, *, #16438, .T. ) ;
#20561=DIRECTION ( 'NONE',  ( -1.000000000000000000, 0.000000000000000000, 0.000000000000000000 ) ) ;
#20562=ADVANCED_FACE ( 'NONE', ( #524 ), #20308, .F. ) ;
#20577=TOROIDAL_SURFACE ( 'NONE', #29517, 38.50000000000000000, 0.9999999999999974465 ) ;
#20596=TOROIDAL_SURFACE ( 'NONE', #6441, 17.50000000000000000, 1.999999999999998224 ) ;
#20597=ORIENTED_EDGE ( 'NONE', *, *, #13398, .T. ) ;
#20598=CARTESIAN_POINT ( 'NONE',  ( 67.49616587369396825, 13.78442380691147839, 47.04930799450051637 ) ) ;
#20605=ADVANCED_FACE ( 'NONE', ( #12705 ), #904, .F. ) ;
#20615=DIRECTION ( 'NONE',  ( -0.000000000000000000, -1.000000000000000000, 0.000000000000000000 ) ) ;
#20617=TOROIDAL_SURFACE ( 'NONE', #2279, 26.49999999999999645, 0.9999999999999956701 ) ;
#20629=CIRCLE ( 'NONE', #14876, 45.93251711706293605 ) ;
#20630=CARTESIAN_POINT ( 'NONE',  ( -18.90214402394280313, 14.86454579224779948, 47.04930799450052348 ) ) ;
#20631=AXIS2_PLACEMENT_3D ( 'NONE', #18886, #26290, #13824 ) ;
#20642=EDGE_CURVE ( 'NONE', #15058, #19572, #22933, .T. ) ;
#20649=DIRECTION ( 'NONE',  ( -0.000000000000000000, -1.000000000000000000, 0.000000000000000000 ) ) ;
#20664=DIRECTION ( 'NONE',  ( -1.000000000000000000, 0.000000000000000000, 0.000000000000000000 ) ) ;
#20684=CARTESIAN_POINT ( 'NONE',  ( -0.9021440239427926944, 14.86454579224779948, 47.04930799450052348 ) ) ;
#20686=DIRECTION ( 'NONE',  ( -0.000000000000000000, -1.000000000000000000, 0.000000000000000000 ) ) ;
#20696=CARTESIAN_POINT ( 'NONE',  ( -14.40214402394279780, 14.86454579224779948, 47.04930799450052348 ) ) ;
#20709=AXIS2_PLACEMENT_3D ( 'NONE', #6196, #6682, #6524 ) ;
#20732=( GEOMETRIC_REPRESENTATION_CONTEXT ( 3 ) GLOBAL_UNCERTAINTY_ASSIGNED_CONTEXT ( ( #14386 ) ) GLOBAL_UNIT_ASSIGNED_CONTEXT ( ( #27772, #10376, #22350 ) ) REPRESENTATION_CONTEXT ( 'NONE', 'WORKASPACE' ) );
#20735=VECTOR ( 'NONE', #6765, 1000.000000000000000 ) ;
#20746=DIRECTION ( 'NONE',  ( 0.000000000000000000, 0.000000000000000000, 1.000000000000000000 ) ) ;
#20760=ADVANCED_FACE ( 'NONE', ( #8247 ), #10884, .F. ) ;
#20762=ORIENTED_EDGE ( 'NONE', *, *, #19844, .F. ) ;
#20794=DIRECTION ( 'NONE',  ( -0.000000000000000000, -1.000000000000000000, 0.000000000000000000 ) ) ;
#20801=ORIENTED_EDGE ( 'NONE', *, *, #20892, .F. ) ;
#20819=ORIENTED_EDGE ( 'NONE', *, *, #13642, .T. ) ;
#20820=DIRECTION ( 'NONE',  ( -0.000000000000000000, -1.000000000000000000, 0.000000000000000000 ) ) ;
#20823=FACE_OUTER_BOUND ( 'NONE', #27875, .T. ) ;
#20829=PLANE ( 'NONE',  #23548 ) ;
#20831=AXIS2_PLACEMENT_3D ( 'NONE', #13219, #7797, #18271 ) ;
#20839=ORIENTED_EDGE ( 'NONE', *, *, #22374, .F. ) ;
#20842=PLANE ( 'NONE',  #7864 ) ;
#20851=ORIENTED_EDGE ( 'NONE', *, *, #29021, .T. ) ;
#20858=DIRECTION ( 'NONE',  ( 0.000000000000000000, 0.000000000000000000, 1.000000000000000000 ) ) ;
#20859=DIRECTION ( 'NONE',  ( -1.000000000000000000, 0.000000000000000000, 0.000000000000000000 ) ) ;
#20873=CIRCLE ( 'NONE', #25583, 31.00000000000000000 ) ;
#20878=ORIENTED_EDGE ( 'NONE', *, *, #12545, .F. ) ;
#20892=EDGE_CURVE ( 'NONE', #22237, #10875, #32391, .T. ) ;
#20899=CARTESIAN_POINT ( 'NONE',  ( 21.09785597605720753, -5.098646251524523443, 47.04930799450052348 ) ) ;
#20900=FACE_OUTER_BOUND ( 'NONE', #26548, .T. ) ;
#20905=DIRECTION ( 'NONE',  ( -1.000000000000000000, 0.000000000000000000, 0.000000000000000000 ) ) ;
#20916=AXIS2_PLACEMENT_3D ( 'NONE', #14925, #24938, #24770 ) ;
#20919=CIRCLE ( 'NONE', #26690, 13.81487396812510937 ) ;
#20949=ORIENTED_EDGE ( 'NONE', *, *, #3259, .T. ) ;
#20950=DIRECTION ( 'NONE',  ( -1.224646799147353207E-16, 0.000000000000000000, -1.000000000000000000 ) ) ;
#20958=VECTOR ( 'NONE', #8434, 1000.000000000000114 ) ;
#20964=EDGE_CURVE ( 'NONE', #16293, #18953, #10392, .T. ) ;
#20980=CARTESIAN_POINT ( 'NONE',  ( 7.596071960694297687, 16.03967147762301693, 47.04930799450052348 ) ) ;
#20997=ADVANCED_FACE ( 'NONE', ( #18839 ), #27145, .T. ) ;
#20998=AXIS2_PLACEMENT_3D ( 'NONE', #23416, #10796, #13098 ) ;
#21001=CARTESIAN_POINT ( 'NONE',  ( 75.19785597605721250, 14.36454579224779948, 47.04930799450052348 ) ) ;
#21008=ORIENTED_EDGE ( 'NONE', *, *, #12647, .T. ) ;
#21011=DIRECTION ( 'NONE',  ( -0.000000000000000000, -1.000000000000000000, 0.000000000000000000 ) ) ;
#21014=AXIS2_PLACEMENT_3D ( 'NONE', #31403, #6125, #23998 ) ;
#21019=CARTESIAN_POINT ( 'NONE',  ( 21.09785597605720753, 14.36454579224779948, 47.04930799450052348 ) ) ;
#21020=CARTESIAN_POINT ( 'NONE',  ( 21.09785597605720753, 14.86454579224779948, 47.04930799450052348 ) ) ;
#21024=EDGE_CURVE ( 'NONE', #7765, #7100, #26729, .T. ) ;
#21038=DIRECTION ( 'NONE',  ( -0.000000000000000000, -1.000000000000000000, 0.000000000000000000 ) ) ;
#21046=DIRECTION ( 'NONE',  ( 0.000000000000000000, 0.000000000000000000, 1.000000000000000000 ) ) ;
#21047=CARTESIAN_POINT ( 'NONE',  ( -12.90214402394279603, 14.86454579224779948, 47.04930799450052348 ) ) ;
#21052=DIRECTION ( 'NONE',  ( -1.000000000000000000, 0.000000000000000000, 0.000000000000000000 ) ) ;
#21070=ORIENTED_EDGE ( 'NONE', *, *, #31836, .T. ) ;
#21078=CIRCLE ( 'NONE', #19509, 25.50000000000000355 ) ;
#21086=CARTESIAN_POINT ( 'NONE',  ( -6.402144023942783591, 13.86454579224779948, 47.04930799450052348 ) ) ;
#21091=VERTEX_POINT ( 'NONE', #8150 ) ;
#21099=TOROIDAL_SURFACE ( 'NONE', #2765, 46.39830989763677849, 0.4000000000000020206 ) ;
#21102=DIRECTION ( 'NONE',  ( -1.000000000000000000, 0.000000000000000000, 0.000000000000000000 ) ) ;
#21113=ORIENTED_EDGE ( 'NONE', *, *, #28074, .F. ) ;
#21118=ORIENTED_EDGE ( 'NONE', *, *, #15453, .T. ) ;
#21122=DIRECTION ( 'NONE',  ( -0.000000000000000000, -1.000000000000000000, 0.000000000000000000 ) ) ;
#21127=FACE_OUTER_BOUND ( 'NONE', #25161, .T. ) ;
#21134=ORIENTED_EDGE ( 'NONE', *, *, #22890, .T. ) ;
#21142=DIRECTION ( 'NONE',  ( -0.000000000000000000, -1.000000000000000000, 0.000000000000000000 ) ) ;
#21149=ADVANCED_FACE ( 'NONE', ( #16008 ), #31118, .F. ) ;
#21151=CIRCLE ( 'NONE', #11728, 54.30000000000000426 ) ;
#21185=VECTOR ( 'NONE', #9800, 1000.000000000000000 ) ;
#21186=ADVANCED_FACE ( 'NONE', ( #28491 ), #13037, .F. ) ;
#21207=CARTESIAN_POINT ( 'NONE',  ( 21.09785597605720753, 14.86454579224779948, 47.04930799450052348 ) ) ;
#21226=DIRECTION ( 'NONE',  ( -1.000000000000000000, 0.000000000000000000, 0.000000000000000000 ) ) ;
#21239=CARTESIAN_POINT ( 'NONE',  ( 21.09785597605720753, 14.86454579224779948, 47.04930799450052348 ) ) ;
#21246=DIRECTION ( 'NONE',  ( -0.000000000000000000, -1.000000000000000000, 0.000000000000000000 ) ) ;
#21249=EDGE_CURVE ( 'NONE', #1796, #18652, #4636, .T. ) ;
#21263=CARTESIAN_POINT ( 'NONE',  ( 53.59785597605720397, 13.86454579224779948, 47.04930799450051637 ) ) ;
#21270=ORIENTED_EDGE ( 'NONE', *, *, #17818, .F. ) ;
#21277=DIRECTION ( 'NONE',  ( -1.000000000000000000, 0.000000000000000000, 0.000000000000000000 ) ) ;
#21296=FACE_OUTER_BOUND ( 'NONE', #12099, .T. ) ;
#21306=DIRECTION ( 'NONE',  ( -1.000000000000000000, 0.000000000000000000, 0.000000000000000000 ) ) ;
#21322=EDGE_CURVE ( 'NONE', #18056, #26091, #30332, .T. ) ;
#21333=ORIENTED_EDGE ( 'NONE', *, *, #7122, .F. ) ;
#21342=VERTEX_POINT ( 'NONE', #2841 ) ;
#21355=CARTESIAN_POINT ( 'NONE',  ( 21.09785597605720753, 13.66454579224780019, 47.04930799450052348 ) ) ;
#21368=CARTESIAN_POINT ( 'NONE',  ( 3.597855976057204419, 14.86454579224779948, 47.04930799450052348 ) ) ;
#21369=AXIS2_PLACEMENT_3D ( 'NONE', #23174, #2824, #30407 ) ;
#21378=DIRECTION ( 'NONE',  ( -0.000000000000000000, -1.000000000000000000, 0.000000000000000000 ) ) ;
#21381=DIRECTION ( 'NONE',  ( -1.000000000000000000, 0.000000000000000000, 0.000000000000000000 ) ) ;
#21382=ORIENTED_EDGE ( 'NONE', *, *, #24984, .F. ) ;
#21391=AXIS2_PLACEMENT_3D ( 'NONE', #13271, #20794, #30817 ) ;
#21399=DIRECTION ( 'NONE',  ( -0.000000000000000000, -1.000000000000000000, 0.000000000000000000 ) ) ;
#21411=DIRECTION ( 'NONE',  ( -0.000000000000000000, -1.000000000000000000, 0.000000000000000000 ) ) ;
#21413=ORIENTED_EDGE ( 'NONE', *, *, #17649, .F. ) ;
#21419=AXIS2_PLACEMENT_3D ( 'NONE', #9178, #25206, #26896 ) ;
#21420=CARTESIAN_POINT ( 'NONE',  ( -22.40214402394279247, 13.86454579224779948, 47.04930799450052348 ) ) ;
#21425=ORIENTED_EDGE ( 'NONE', *, *, #20380, .T. ) ;
#21440=DIRECTION ( 'NONE',  ( -0.000000000000000000, -1.000000000000000000, 0.000000000000000000 ) ) ;
#21465=ORIENTED_EDGE ( 'NONE', *, *, #20041, .F. ) ;
#21486=( LENGTH_UNIT ( ) NAMED_UNIT ( * ) SI_UNIT ( .MILLI., .METRE. ) );
#21494=ORIENTED_EDGE ( 'NONE', *, *, #2228, .F. ) ;
#21509=AXIS2_PLACEMENT_3D ( 'NONE', #10216, #13005, #22837 ) ;
#21515=FACE_OUTER_BOUND ( 'NONE', #4036, .T. ) ;
#21535=CARTESIAN_POINT ( 'NONE',  ( -18.40214402394279603, 14.86454579224779948, 47.04930799450052348 ) ) ;
#21563=DIRECTION ( 'NONE',  ( -0.000000000000000000, -1.000000000000000000, 0.000000000000000000 ) ) ;
#21565=EDGE_LOOP ( 'NONE', ( #20420, #22234, #29902, #7340 ) ) ;
#21578=ORIENTED_EDGE ( 'NONE', *, *, #2929, .T. ) ;
#21580=DIRECTION ( 'NONE',  ( -1.224646799147353207E-16, 0.000000000000000000, -1.000000000000000000 ) ) ;
#21593=EDGE_LOOP ( 'NONE', ( #9666, #31361, #22525, #26050 ) ) ;
#21598=ADVANCED_FACE ( 'NONE', ( #21515 ), #25411, .T. ) ;
#21601=CARTESIAN_POINT ( 'NONE',  ( 7.896202261960366009, 17.36467600858027183, 47.04930799450052348 ) ) ;
#21612=ORIENTED_EDGE ( 'NONE', *, *, #30344, .F. ) ;
#21627=CARTESIAN_POINT ( 'NONE',  ( 21.09785597605720753, 17.36467600858027183, 47.04930799450052348 ) ) ;
#21628=LINE ( 'NONE', #19651, #23477 ) ;
#21634=ORIENTED_EDGE ( 'NONE', *, *, #29393, .F. ) ;
#21637=CARTESIAN_POINT ( 'NONE',  ( 67.77233896511883415, 13.66454579224780019, 47.04930799450051637 ) ) ;
#21644=AXIS2_PLACEMENT_3D ( 'NONE', #160, #319, #18036 ) ;
#21697=ORIENTED_EDGE ( 'NONE', *, *, #19784, .F. ) ;
#21710=DIRECTION ( 'NONE',  ( -0.000000000000000000, -1.000000000000000000, 0.000000000000000000 ) ) ;
#21717=CIRCLE ( 'NONE', #29055, 0.7905694150420993216 ) ;
#21723=CIRCLE ( 'NONE', #7601, 19.00000000000000000 ) ;
#21725=FACE_OUTER_BOUND ( 'NONE', #30614, .T. ) ;
#21731=DIRECTION ( 'NONE',  ( -1.000000000000000000, 0.000000000000000000, 0.000000000000000000 ) ) ;
#21742=ADVANCED_FACE ( 'NONE', ( #29904 ), #22232, .F. ) ;
#21762=LINE ( 'NONE', #31783, #14583 ) ;
#21785=EDGE_CURVE ( 'NONE', #31872, #16293, #21717, .T. ) ;
#21790=CARTESIAN_POINT ( 'NONE',  ( -20.40214402394279603, 14.86454579224779948, 47.04930799450052348 ) ) ;
#21800=DIRECTION ( 'NONE',  ( -1.000000000000000000, 0.000000000000000000, 0.000000000000000000 ) ) ;
#21801=FACE_OUTER_BOUND ( 'NONE', #3378, .T. ) ;
#21803=AXIS2_PLACEMENT_3D ( 'NONE', #29062, #11671, #6254 ) ;
#21819=ORIENTED_EDGE ( 'NONE', *, *, #12318, .F. ) ;
#21825=ORIENTED_EDGE ( 'NONE', *, *, #19998, .T. ) ;
#21837=CARTESIAN_POINT ( 'NONE',  ( 21.09785597605720753, 13.86454579224779948, 47.04930799450052348 ) ) ;
#21841=CARTESIAN_POINT ( 'NONE',  ( 55.09785597605721108, 13.86454579224779948, 47.04930799450051637 ) ) ;
#21855=DIRECTION ( 'NONE',  ( -1.000000000000000000, 0.000000000000000000, 0.000000000000000000 ) ) ;
#21863=CARTESIAN_POINT ( 'NONE',  ( -9.902144023942794249, -5.098646251524523443, 47.04930799450052348 ) ) ;
#21882=ORIENTED_EDGE ( 'NONE', *, *, #9005, .T. ) ;
#21898=CARTESIAN_POINT ( 'NONE',  ( -25.57662701300441555, 14.36454579224780126, 47.04930799450052348 ) ) ;
#21907=DIRECTION ( 'NONE',  ( -0.000000000000000000, -1.000000000000000000, 0.000000000000000000 ) ) ;
#21926=DIRECTION ( 'NONE',  ( -1.000000000000000000, 0.000000000000000000, 0.000000000000000000 ) ) ;
#21966=AXIS2_PLACEMENT_3D ( 'NONE', #13702, #572, #11081 ) ;
#21971=EDGE_LOOP ( 'NONE', ( #9612, #31617, #27019, #297 ) ) ;
#21978=EDGE_CURVE ( 'NONE', #7331, #13945, #4456, .T. ) ;
#21983=CIRCLE ( 'NONE', #10485, 1.499999999999994449 ) ;
#21990=ORIENTED_EDGE ( 'NONE', *, *, #14354, .T. ) ;
#21993=EDGE_CURVE ( 'NONE', #163, #12910, #15479, .T. ) ;
#21997=AXIS2_PLACEMENT_3D ( 'NONE', #16449, #25980, #31401 ) ;
#22000=ORIENTED_EDGE ( 'NONE', *, *, #20283, .T. ) ;
#22014=DIRECTION ( 'NONE',  ( -1.000000000000000000, 0.000000000000000000, 0.000000000000000000 ) ) ;
#22021=ORIENTED_EDGE ( 'NONE', *, *, #3618, .F. ) ;
#22034=DIRECTION ( 'NONE',  ( -1.000000000000000000, 0.000000000000000000, 0.000000000000000000 ) ) ;
#22038=EDGE_CURVE ( 'NONE', #3892, #24509, #6038, .T. ) ;
#22051=CIRCLE ( 'NONE', #14225, 0.6621856154243876968 ) ;
#22057=FACE_OUTER_BOUND ( 'NONE', #25510, .T. ) ;
#22075=ORIENTED_EDGE ( 'NONE', *, *, #29768, .T. ) ;
#22077=DIRECTION ( 'NONE',  ( 0.9999997877697283100, 0.0006515063303658816165, 0.000000000000000000 ) ) ;
#22078=VECTOR ( 'NONE', #9277, 1000.000000000000000 ) ;
#22086=AXIS2_PLACEMENT_3D ( 'NONE', #9727, #11532, #21855 ) ;
#22089=DIRECTION ( 'NONE',  ( 0.9275012328650849014, -0.3738200944756011057, -1.135861416033450161E-16 ) ) ;
#22100=EDGE_LOOP ( 'NONE', ( #22021, #10899, #5778, #24384 ) ) ;
#22112=CARTESIAN_POINT ( 'NONE',  ( 75.19785597605721250, 14.36454579224779948, 47.04930799450051637 ) ) ;
#22149=VERTEX_POINT ( 'NONE', #23433 ) ;
#22152=LINE ( 'NONE', #16906, #14602 ) ;
#22163=CIRCLE ( 'NONE', #8011, 15.23374605753642186 ) ;
#22165=DIRECTION ( 'NONE',  ( -0.000000000000000000, -1.000000000000000000, 0.000000000000000000 ) ) ;
#22166=DIRECTION ( 'NONE',  ( 0.000000000000000000, 1.000000000000000000, 0.000000000000000000 ) ) ;
#22167=FACE_OUTER_BOUND ( 'NONE', #28562, .T. ) ;
#22190=VERTEX_POINT ( 'NONE', #22940 ) ;
#22204=FACE_OUTER_BOUND ( 'NONE', #24966, .T. ) ;
#22205=EDGE_CURVE ( 'NONE', #4851, #19129, #11799, .T. ) ;
#22207=LINE ( 'NONE', #19738, #27252 ) ;
#22208=CARTESIAN_POINT ( 'NONE',  ( 21.09785597605720753, 15.19538130838178169, 47.04930799450052348 ) ) ;
#22221=ORIENTED_EDGE ( 'NONE', *, *, #15453, .F. ) ;
#22230=DIRECTION ( 'NONE',  ( -1.000000000000000000, 0.000000000000000000, 0.000000000000000000 ) ) ;
#22232=TOROIDAL_SURFACE ( 'NONE', #8102, 26.49999999999999645, 0.9999999999999956701 ) ;
#22234=ORIENTED_EDGE ( 'NONE', *, *, #17407, .T. ) ;
#22237=VERTEX_POINT ( 'NONE', #21601 ) ;
#22241=ORIENTED_EDGE ( 'NONE', *, *, #29805, .F. ) ;
#22245=STYLED_ITEM('',(#32529),#1196);
#22248=AXIS2_PLACEMENT_3D ( 'NONE', #11616, #9804, #14404 ) ;
#22250=EDGE_CURVE ( 'NONE', #14305, #18233, #20873, .T. ) ;
#22261=DIRECTION ( 'NONE',  ( 1.000000000000000000, 0.000000000000000000, 0.000000000000000000 ) ) ;
#22264=ORIENTED_EDGE ( 'NONE', *, *, #32441, .T. ) ;
#22271=DIRECTION ( 'NONE',  ( -0.000000000000000000, -1.000000000000000000, 0.000000000000000000 ) ) ;
#22275=CARTESIAN_POINT ( 'NONE',  ( 21.09785597605720753, 14.61319044934410627, 47.04930799450052348 ) ) ;
#22286=DIRECTION ( 'NONE',  ( -0.000000000000000000, -1.000000000000000000, 0.000000000000000000 ) ) ;
#22301=AXIS2_PLACEMENT_3D ( 'NONE', #3489, #21046, #30759 ) ;
#22310=CARTESIAN_POINT ( 'NONE',  ( 52.09785597605720397, -5.098646251524523443, 47.04930799450051637 ) ) ;
#22322=FACE_BOUND ( 'NONE', #23519, .T. ) ;
#22327=CARTESIAN_POINT ( 'NONE',  ( 21.09785597605720753, 14.86454579224779948, 47.04930799450052348 ) ) ;
#22329=CIRCLE ( 'NONE', #12387, 54.10000000000000142 ) ;
#22336=DIRECTION ( 'NONE',  ( -0.000000000000000000, -1.000000000000000000, 0.000000000000000000 ) ) ;
#22346=CARTESIAN_POINT ( 'NONE',  ( 21.09785597605720753, -5.098646251524523443, 47.04930799450052348 ) ) ;
#22350=( NAMED_UNIT ( * ) SI_UNIT ( $, .STERADIAN. ) SOLID_ANGLE_UNIT ( ) );
#22359=DIRECTION ( 'NONE',  ( -1.000000000000000000, 0.000000000000000000, 0.000000000000000000 ) ) ;
#22369=ORIENTED_EDGE ( 'NONE', *, *, #22374, .T. ) ;
#22374=EDGE_CURVE ( 'NONE', #4784, #13945, #21762, .T. ) ;
#22375=EDGE_CURVE ( 'NONE', #18804, #28622, #12097, .T. ) ;
#22411=ORIENTED_EDGE ( 'NONE', *, *, #31267, .F. ) ;
#22441=ORIENTED_EDGE ( 'NONE', *, *, #6366, .T. ) ;
#22467=DIRECTION ( 'NONE',  ( -0.000000000000000000, -1.000000000000000000, 0.000000000000000000 ) ) ;
#22468=CARTESIAN_POINT ( 'NONE',  ( 21.09785597605720753, 14.86454579224779948, 47.04930799450052348 ) ) ;
#22482=DIRECTION ( 'NONE',  ( -1.000000000000000000, 0.000000000000000000, 0.000000000000000000 ) ) ;
#22488=TOROIDAL_SURFACE ( 'NONE', #32474, 26.49999999999999645, 1.499999999999997780 ) ;
#22491=EDGE_LOOP ( 'NONE', ( #15283, #30243, #9133, #25655 ) ) ;
#22519=ORIENTED_EDGE ( 'NONE', *, *, #17705, .T. ) ;
#22520=CARTESIAN_POINT ( 'NONE',  ( 40.09785597605721108, 13.86454579224779948, 47.04930799450052348 ) ) ;
#22525=ORIENTED_EDGE ( 'NONE', *, *, #8803, .T. ) ;
#22534=CIRCLE ( 'NONE', #11518, 0.5000000000000004441 ) ;
#22566=ADVANCED_FACE ( 'NONE', ( #23396 ), #25375, .T. ) ;
#22568=EDGE_CURVE ( 'NONE', #29739, #163, #4088, .T. ) ;
#22582=ORIENTED_EDGE ( 'NONE', *, *, #30472, .F. ) ;
#22587=DIRECTION ( 'NONE',  ( -1.000000000000000000, 0.000000000000000000, 0.000000000000000000 ) ) ;
#22615=CARTESIAN_POINT ( 'NONE',  ( 21.09785597605720753, 13.86454579224779948, 47.04930799450052348 ) ) ;
#22619=AXIS2_PLACEMENT_3D ( 'NONE', #9613, #9937, #15029 ) ;
#22642=DIRECTION ( 'NONE',  ( 0.000000000000000000, 1.000000000000000000, 0.000000000000000000 ) ) ;
#22652=CYLINDRICAL_SURFACE ( 'NONE', #6781, 43.50000000000000000 ) ;
#22665=DIRECTION ( 'NONE',  ( -0.000000000000000000, -1.000000000000000000, 0.000000000000000000 ) ) ;
#22719=CARTESIAN_POINT ( 'NONE',  ( 21.09785597605720753, 13.86454579224779948, 47.04930799450052348 ) ) ;
#22746=EDGE_CURVE ( 'NONE', #12393, #17230, #956, .T. ) ;
#22754=CARTESIAN_POINT ( 'NONE',  ( -5.402144023942789808, 13.86454579224779948, 47.04930799450052348 ) ) ;
#22762=CYLINDRICAL_SURFACE ( 'NONE', #1585, 19.50000000000000000 ) ;
#22768=ORIENTED_EDGE ( 'NONE', *, *, #20266, .T. ) ;
#22777=AXIS2_PLACEMENT_3D ( 'NONE', #5102, #24963, #17079 ) ;
#22788=CARTESIAN_POINT ( 'NONE',  ( -17.40214402394279247, 13.86454579224779948, 47.04930799450052348 ) ) ;
#22800=CARTESIAN_POINT ( 'NONE',  ( 21.09785597605720753, 13.86454579224779948, 47.04930799450052348 ) ) ;
#22815=LINE ( 'NONE', #10521, #9170 ) ;
#22817=AXIS2_PLACEMENT_3D ( 'NONE', #4061, #9154, #13770 ) ;
#22820=AXIS2_PLACEMENT_3D ( 'NONE', #8260, #1023, #5633 ) ;
#22824=DIRECTION ( 'NONE',  ( -0.000000000000000000, -1.000000000000000000, 0.000000000000000000 ) ) ;
#22830=CARTESIAN_POINT ( 'NONE',  ( -0.4021440239427888086, 13.86454579224779948, 47.04930799450052348 ) ) ;
#22837=DIRECTION ( 'NONE',  ( -1.000000000000000000, 0.000000000000000000, 0.000000000000000000 ) ) ;
#22838=FACE_OUTER_BOUND ( 'NONE', #2350, .T. ) ;
#22852=ADVANCED_FACE ( 'NONE', ( #17581 ), #18256, .T. ) ;
#22881=ORIENTED_EDGE ( 'NONE', *, *, #12647, .F. ) ;
#22883=CARTESIAN_POINT ( 'NONE',  ( 21.09785597605720753, 14.16454579224779842, 47.04930799450052348 ) ) ;
#22885=DIRECTION ( 'NONE',  ( -0.000000000000000000, -1.000000000000000000, 0.000000000000000000 ) ) ;
#22890=EDGE_CURVE ( 'NONE', #24509, #490, #10408, .T. ) ;
#22907=CIRCLE ( 'NONE', #19742, 31.00000000000000000 ) ;
#22920=LINE ( 'NONE', #8163, #4741 ) ;
#22933=CIRCLE ( 'NONE', #16621, 2.000000000000001776 ) ;
#22935=ORIENTED_EDGE ( 'NONE', *, *, #24008, .T. ) ;
#22936=ADVANCED_FACE ( 'NONE', ( #29373 ), #16716, .T. ) ;
#22940=CARTESIAN_POINT ( 'NONE',  ( 55.09785597605721108, 14.86454579224779948, 47.04930799450051637 ) ) ;
#22941=ORIENTED_EDGE ( 'NONE', *, *, #32441, .F. ) ;
#22946=VERTEX_POINT ( 'NONE', #19511 ) ;
#22950=ORIENTED_EDGE ( 'NONE', *, *, #21322, .F. ) ;
#22973=EDGE_CURVE ( 'NONE', #18982, #31760, #18765, .T. ) ;
#23003=CYLINDRICAL_SURFACE ( 'NONE', #14486, 27.99999999999999645 ) ;
#23021=CARTESIAN_POINT ( 'NONE',  ( 7.282982007932096380, 15.57592086119046826, 47.04930799450052348 ) ) ;
#23029=ORIENTED_EDGE ( 'NONE', *, *, #30440, .T. ) ;
#23034=AXIS2_PLACEMENT_3D ( 'NONE', #22615, #10155, #20149 ) ;
#23037=ORIENTED_EDGE ( 'NONE', *, *, #20380, .F. ) ;
#23041=DIRECTION ( 'NONE',  ( -0.000000000000000000, -1.000000000000000000, 0.000000000000000000 ) ) ;
#23043=DIRECTION ( 'NONE',  ( -1.000000000000000000, 0.000000000000000000, 0.000000000000000000 ) ) ;
#23060=CIRCLE ( 'NONE', #25692, 0.7905694150421027633 ) ;
#23066=EDGE_CURVE ( 'NONE', #12208, #31745, #27716, .T. ) ;
#23070=AXIS2_PLACEMENT_3D ( 'NONE', #11215, #31243, #8742 ) ;
#23073=DIRECTION ( 'NONE',  ( -1.000000000000000000, 0.000000000000000000, 0.000000000000000000 ) ) ;
#23083=CARTESIAN_POINT ( 'NONE',  ( 5.092160267343103897, 14.99513937955032716, 47.04930799450052348 ) ) ;
#23113=CIRCLE ( 'NONE', #5300, 13.50178401536290806 ) ;
#23122=DIRECTION ( 'NONE',  ( -1.000000000000000000, 0.000000000000000000, 0.000000000000000000 ) ) ;
#23130=ADVANCED_FACE ( 'NONE', ( #17870 ), #30030, .F. ) ;
#23162=CARTESIAN_POINT ( 'NONE',  ( 75.19785597605721250, 14.86454579224779948, 47.04930799450051637 ) ) ;
#23168=DIRECTION ( 'NONE',  ( 1.000000000000000000, 0.000000000000000000, 0.000000000000000000 ) ) ;
#23174=CARTESIAN_POINT ( 'NONE',  ( 21.09785597605720753, 14.86454579224779948, 47.04930799450052348 ) ) ;
#23190=ADVANCED_FACE ( 'NONE', ( #7546 ), #17541, .F. ) ;
#23207=EDGE_CURVE ( 'NONE', #28560, #10403, #5186, .T. ) ;
#23255=DIRECTION ( 'NONE',  ( -1.000000000000000000, 0.000000000000000000, 0.000000000000000000 ) ) ;
#23262=ORIENTED_EDGE ( 'NONE', *, *, #20283, .F. ) ;
#23265=DIRECTION ( 'NONE',  ( -1.000000000000000000, 0.000000000000000000, 0.000000000000000000 ) ) ;
#23289=VERTEX_POINT ( 'NONE', #6848 ) ;
#23312=TOROIDAL_SURFACE ( 'NONE', #10226, 15.27594751018003194, 0.2551199516247882326 ) ;
#23318=CARTESIAN_POINT ( 'NONE',  ( 67.84785597605720397, 13.61454579224779771, 47.04930799450051637 ) ) ;
#23343=AXIS2_PLACEMENT_3D ( 'NONE', #10830, #20820, #30844 ) ;
#23352=ORIENTED_EDGE ( 'NONE', *, *, #14028, .F. ) ;
#23387=TOROIDAL_SURFACE ( 'NONE', #6095, 13.20178401536290913, 0.2000000000000002609 ) ;
#23388=ORIENTED_EDGE ( 'NONE', *, *, #17675, .T. ) ;
#23396=FACE_OUTER_BOUND ( 'NONE', #16442, .T. ) ;
#23416=CARTESIAN_POINT ( 'NONE',  ( 21.09785597605720753, 13.86454579224779948, 47.04930799450052348 ) ) ;
#23421=CARTESIAN_POINT ( 'NONE',  ( 43.09785597605719687, 13.86454579224779948, 47.04930799450052348 ) ) ;
#23433=CARTESIAN_POINT ( 'NONE',  ( 36.62540880027166423, 15.19538130838178169, 47.04930799450052348 ) ) ;
#23434=CIRCLE ( 'NONE', #20518, 0.1999999999999987899 ) ;
#23441=EDGE_LOOP ( 'NONE', ( #11251, #12088, #25545, #8953 ) ) ;
#23477=VECTOR ( 'NONE', #27378, 1000.000000000000000 ) ;
#23492=FACE_OUTER_BOUND ( 'NONE', #16086, .T. ) ;
#23503=AXIS2_PLACEMENT_3D ( 'NONE', #15684, #27960, #30263 ) ;
#23507=AXIS2_PLACEMENT_3D ( 'NONE', #25557, #20950, #617 ) ;
#23519=EDGE_LOOP ( 'NONE', ( #22000, #20259 ) ) ;
#23541=VERTEX_POINT ( 'NONE', #21086 ) ;
#23548=AXIS2_PLACEMENT_3D ( 'NONE', #28390, #7722, #15579 ) ;
#23563=CARTESIAN_POINT ( 'NONE',  ( 21.09785597605720753, 13.86454579224779948, 47.04930799450052348 ) ) ;
#23585=CIRCLE ( 'NONE', #8904, 1.500000000000001332 ) ;
#23595=TOROIDAL_SURFACE ( 'NONE', #5267, 23.50000000000000000, 1.500000000000001332 ) ;
#23605=ORIENTED_EDGE ( 'NONE', *, *, #13398, .F. ) ;
#23617=DIRECTION ( 'NONE',  ( -1.000000000000000000, 0.000000000000000000, 0.000000000000000000 ) ) ;
#23629=TOROIDAL_SURFACE ( 'NONE', #9461, 17.50000000000000000, 1.499999999999998668 ) ;
#23639=ADVANCED_FACE ( 'NONE', ( #18778 ), #26663, .T. ) ;
#23642=CARTESIAN_POINT ( 'NONE',  ( 49.09785597605720397, -5.098646251524523443, 47.04930799450052348 ) ) ;
#23643=CARTESIAN_POINT ( 'NONE',  ( 21.09785597605720753, 14.46497581658974063, 47.04930799450052348 ) ) ;
#23650=CIRCLE ( 'NONE', #7918, 45.93251711706293605 ) ;
#23655=ORIENTED_EDGE ( 'NONE', *, *, #29021, .F. ) ;
#23673=AXIS2_PLACEMENT_3D ( 'NONE', #9566, #7097, #17098 ) ;
#23675=EDGE_CURVE ( 'NONE', #12822, #15058, #2061, .T. ) ;
#23681=FACE_OUTER_BOUND ( 'NONE', #25789, .T. ) ;
#23711=VECTOR ( 'NONE', #22467, 1000.000000000000000 ) ;
#23718=DIRECTION ( 'NONE',  ( -0.000000000000000000, -1.000000000000000000, 0.000000000000000000 ) ) ;
#23737=EDGE_LOOP ( 'NONE', ( #12258, #16028, #26504, #8653 ) ) ;
#23740=EDGE_LOOP ( 'NONE', ( #27168, #30290, #31890, #26001 ) ) ;
#23744=ADVANCED_FACE ( 'NONE', ( #19264 ), #25682, .T. ) ;
#23748=TOROIDAL_SURFACE ( 'NONE', #4877, 38.50000000000000000, 0.9999999999999974465 ) ;
#23752=AXIS2_PLACEMENT_3D ( 'NONE', #5021, #27656, #2393 ) ;
#23755=CARTESIAN_POINT ( 'NONE',  ( 21.09785597605720753, 13.86454579224779948, 47.04930799450052348 ) ) ;
#23765=CARTESIAN_POINT ( 'NONE',  ( 21.09785597605720753, 14.86454579224779948, 47.04930799450052348 ) ) ;
#23790=DIRECTION ( 'NONE',  ( -0.000000000000000000, -1.000000000000000000, 0.000000000000000000 ) ) ;
#23805=CARTESIAN_POINT ( 'NONE',  ( -10.40214402394279425, 14.86454579224779948, 47.04930799450052348 ) ) ;
#23825=EDGE_CURVE ( 'NONE', #26196, #12159, #22534, .T. ) ;
#23832=CARTESIAN_POINT ( 'NONE',  ( 66.59450633559774246, 13.78276522714992147, 47.04930799450051637 ) ) ;
#23833=ORIENTED_EDGE ( 'NONE', *, *, #30721, .F. ) ;
#23849=DIRECTION ( 'NONE',  ( -1.000000000000000000, 0.000000000000000000, 0.000000000000000000 ) ) ;
#23850=EDGE_LOOP ( 'NONE', ( #8674, #32130, #29657, #14407 ) ) ;
#23856=FACE_OUTER_BOUND ( 'NONE', #23441, .T. ) ;
#23866=VECTOR ( 'NONE', #7547, 1000.000000000000000 ) ;
#23869=AXIS2_PLACEMENT_3D ( 'NONE', #21207, #26146, #21052 ) ;
#23876=ORIENTED_EDGE ( 'NONE', *, *, #22746, .F. ) ;
#23877=DIRECTION ( 'NONE',  ( -0.000000000000000000, -1.000000000000000000, 0.000000000000000000 ) ) ;
#23895=ORIENTED_EDGE ( 'NONE', *, *, #5049, .F. ) ;
#23896=DIRECTION ( 'NONE',  ( 0.000000000000000000, 0.000000000000000000, 1.000000000000000000 ) ) ;
#23908=CIRCLE ( 'NONE', #13959, 13.81487396812510937 ) ;
#23915=FACE_OUTER_BOUND ( 'NONE', #15047, .T. ) ;
#23918=VERTEX_POINT ( 'NONE', #2045 ) ;
#23946=VERTEX_POINT ( 'NONE', #30603 ) ;
#23970=EDGE_CURVE ( 'NONE', #31321, #18652, #15497, .T. ) ;
#23972=ORIENTED_EDGE ( 'NONE', *, *, #23675, .F. ) ;
#23981=AXIS2_PLACEMENT_3D ( 'NONE', #1281, #18196, #28227 ) ;
#23985=CARTESIAN_POINT ( 'NONE',  ( 21.09785597605720753, 13.86454579224779948, 47.04930799450052348 ) ) ;
#23998=DIRECTION ( 'NONE',  ( -1.000000000000000000, 0.000000000000000000, 0.000000000000000000 ) ) ;
#24008=EDGE_CURVE ( 'NONE', #5510, #20520, #21983, .T. ) ;
#24020=ORIENTED_EDGE ( 'NONE', *, *, #16438, .F. ) ;
#24048=DIRECTION ( 'NONE',  ( -0.000000000000000000, -1.000000000000000000, 0.000000000000000000 ) ) ;
#24052=DIRECTION ( 'NONE',  ( -1.224646799147353207E-16, 0.000000000000000000, -1.000000000000000000 ) ) ;
#24059=ORIENTED_EDGE ( 'NONE', *, *, #4708, .F. ) ;
#24066=CARTESIAN_POINT ( 'NONE',  ( 21.09785597605720753, 14.86454579224779948, 47.04930799450052348 ) ) ;
#24073=DIRECTION ( 'NONE',  ( -1.000000000000000000, 0.000000000000000000, 0.000000000000000000 ) ) ;
#24083=CIRCLE ( 'NONE', #492, 13.30165371409683850 ) ;
#24095=CARTESIAN_POINT ( 'NONE',  ( 21.09785597605720753, 14.86454579224779948, 47.04930799450052348 ) ) ;
#24139=DIRECTION ( 'NONE',  ( 0.000000000000000000, 0.000000000000000000, 1.000000000000000000 ) ) ;
#24145=CIRCLE ( 'NONE', #29406, 25.00000000000000000 ) ;
#24168=AXIS2_PLACEMENT_3D ( 'NONE', #24980, #12354, #17915 ) ;
#24175=CARTESIAN_POINT ( 'NONE',  ( 21.09785597605720753, -5.098646251524523443, 47.04930799450052348 ) ) ;
#24219=ORIENTED_EDGE ( 'NONE', *, *, #27109, .T. ) ;
#24229=ADVANCED_FACE ( 'NONE', ( #6124 ), #25701, .F. ) ;
#24230=ORIENTED_EDGE ( 'NONE', *, *, #7356, .T. ) ;
#24231=CIRCLE ( 'NONE', #9025, 22.00000000000000000 ) ;
#24261=DIRECTION ( 'NONE',  ( -1.000000000000000000, 0.000000000000000000, 0.000000000000000000 ) ) ;
#24263=ORIENTED_EDGE ( 'NONE', *, *, #6366, .F. ) ;
#24271=ORIENTED_EDGE ( 'NONE', *, *, #18576, .F. ) ;
#24273=CIRCLE ( 'NONE', #28480, 2.000000000000001776 ) ;
#24283=CARTESIAN_POINT ( 'NONE',  ( 21.09785597605720753, 14.86454579224779948, 47.04930799450052348 ) ) ;
#24295=DIRECTION ( 'NONE',  ( -1.000000000000000000, 0.000000000000000000, 0.000000000000000000 ) ) ;
#24317=DIRECTION ( 'NONE',  ( 0.000000000000000000, 0.000000000000000000, 1.000000000000000000 ) ) ;
#24384=ORIENTED_EDGE ( 'NONE', *, *, #23970, .F. ) ;
#24390=VECTOR ( 'NONE', #28127, 1000.000000000000000 ) ;
#24407=CIRCLE ( 'NONE', #15490, 31.00000000000000000 ) ;
#24442=EDGE_CURVE ( 'NONE', #31760, #17055, #24145, .T. ) ;
#24445=( NAMED_UNIT ( * ) SI_UNIT ( $, .STERADIAN. ) SOLID_ANGLE_UNIT ( ) );
#24455=FACE_OUTER_BOUND ( 'NONE', #19735, .T. ) ;
#24482=EDGE_CURVE ( 'NONE', #2557, #10177, #15769, .T. ) ;
#24498=DIRECTION ( 'NONE',  ( -1.000000000000000000, 0.000000000000000000, 0.000000000000000000 ) ) ;
#24509=VERTEX_POINT ( 'NONE', #18072 ) ;
#24511=ORIENTED_EDGE ( 'NONE', *, *, #126, .F. ) ;
#24514=EDGE_LOOP ( 'NONE', ( #24521, #9642, #22941, #1537 ) ) ;
#24519=AXIS2_PLACEMENT_3D ( 'NONE', #8465, #15852, #18462 ) ;
#24521=ORIENTED_EDGE ( 'NONE', *, *, #31648, .T. ) ;
#24522=CYLINDRICAL_SURFACE ( 'NONE', #25962, 19.00000000000000000 ) ;
#24535=TOROIDAL_SURFACE ( 'NONE', #19296, 13.50178401536290806, 0.5000000000000002220 ) ;
#24537=CARTESIAN_POINT ( 'NONE',  ( 21.09785597605720753, -5.098646251524523443, 47.04930799450052348 ) ) ;
#24539=CARTESIAN_POINT ( 'NONE',  ( 21.09785597605720753, -5.098646251524523443, 47.04930799450052348 ) ) ;
#24548=CIRCLE ( 'NONE', #9348, 43.00000000000000000 ) ;
#24606=CIRCLE ( 'NONE', #5224, 43.00000000000000000 ) ;
#24614=CARTESIAN_POINT ( 'NONE',  ( 21.09785597605720753, 13.86454579224779948, 47.04930799450052348 ) ) ;
#24631=CARTESIAN_POINT ( 'NONE',  ( 21.09785597605720753, 17.36467600858027183, 47.04930799450052348 ) ) ;
#24634=CARTESIAN_POINT ( 'NONE',  ( 42.59785597605720397, 14.86454579224779948, 47.04930799450052348 ) ) ;
#24639=EDGE_CURVE ( 'NONE', #17931, #10875, #31496, .T. ) ;
#24654=CARTESIAN_POINT ( 'NONE',  ( -11.40214402394279603, 13.86454579224779948, 47.04930799450052348 ) ) ;
#24657=AXIS2_PLACEMENT_3D ( 'NONE', #22468, #6111, #2621 ) ;
#24668=FACE_OUTER_BOUND ( 'NONE', #2912, .T. ) ;
#24672=VERTEX_POINT ( 'NONE', #9152 ) ;
#24704=FACE_OUTER_BOUND ( 'NONE', #26299, .T. ) ;
#24747=TOROIDAL_SURFACE ( 'NONE', #18962, 46.75000000000000000, 0.7905694150421007649 ) ;
#24758=CIRCLE ( 'NONE', #31576, 25.50000000000000355 ) ;
#24763=PRODUCT_DEFINITION_SHAPE ( 'NONE', 'NONE',  #8511 ) ;
#24770=DIRECTION ( 'NONE',  ( -1.000000000000000000, 0.000000000000000000, 0.000000000000000000 ) ) ;
#24788=DIRECTION ( 'NONE',  ( -1.000000000000000000, 0.000000000000000000, 0.000000000000000000 ) ) ;
#24844=CARTESIAN_POINT ( 'NONE',  ( 21.09785597605720753, 14.86454579224779948, 47.04930799450052348 ) ) ;
#24857=CARTESIAN_POINT ( 'NONE',  ( 34.09963999142011204, 17.16467605102632632, 47.04930799450052348 ) ) ;
#24872=DIRECTION ( 'NONE',  ( -0.000000000000000000, -1.000000000000000000, 0.000000000000000000 ) ) ;
#24876=DIRECTION ( 'NONE',  ( -1.000000000000000000, 0.000000000000000000, 0.000000000000000000 ) ) ;
#24899=DIRECTION ( 'NONE',  ( -0.000000000000000000, -1.000000000000000000, 0.000000000000000000 ) ) ;
#24913=EDGE_CURVE ( 'NONE', #12822, #23541, #17095, .T. ) ;
#24918=CONICAL_SURFACE ( 'NONE', #1845, 13.81487396812510937, 1.187672012580059944 ) ;
#24937=ORIENTED_EDGE ( 'NONE', *, *, #23825, .T. ) ;
#24938=DIRECTION ( 'NONE',  ( -0.000000000000000000, -1.000000000000000000, 0.000000000000000000 ) ) ;
#24943=ORIENTED_EDGE ( 'NONE', *, *, #28574, .T. ) ;
#24944=DIRECTION ( 'NONE',  ( -0.000000000000000000, -1.000000000000000000, 0.000000000000000000 ) ) ;
#24960=ORIENTED_EDGE ( 'NONE', *, *, #12778, .F. ) ;
#24963=DIRECTION ( 'NONE',  ( -0.000000000000000000, -1.000000000000000000, 0.000000000000000000 ) ) ;
#24964=AXIS2_PLACEMENT_3D ( 'NONE', #4833, #9919, #29779 ) ;
#24966=EDGE_LOOP ( 'NONE', ( #27852, #21825, #8924, #26535 ) ) ;
#24975=EDGE_CURVE ( 'NONE', #16293, #25493, #13192, .T. ) ;
#24980=CARTESIAN_POINT ( 'NONE',  ( 21.09785597605720753, 14.98269195386757602, 47.04930799450052348 ) ) ;
#24984=EDGE_CURVE ( 'NONE', #12804, #10005, #1120, .T. ) ;
#24987=ADVANCED_FACE ( 'NONE', ( #9883 ), #20365, .F. ) ;
#25017=ORIENTED_EDGE ( 'NONE', *, *, #29126, .F. ) ;
#25057=CARTESIAN_POINT ( 'NONE',  ( -2.402144023942794249, 14.86454579224779948, 47.04930799450052348 ) ) ;
#25070=CARTESIAN_POINT ( 'NONE',  ( 21.09785597605720753, 13.86454579224779948, 47.04930799450052348 ) ) ;
#25078=ORIENTED_EDGE ( 'NONE', *, *, #17154, .T. ) ;
#25089=ORIENTED_EDGE ( 'NONE', *, *, #23207, .F. ) ;
#25124=AXIS2_PLACEMENT_3D ( 'NONE', #27560, #2608, #148 ) ;
#25131=AXIS2_PLACEMENT_3D ( 'NONE', #22327, #22165, #6911 ) ;
#25133=DIRECTION ( 'NONE',  ( -1.000000000000000000, 0.000000000000000000, 0.000000000000000000 ) ) ;
#25161=EDGE_LOOP ( 'NONE', ( #22950, #14562, #20552, #25584 ) ) ;
#25167=CARTESIAN_POINT ( 'NONE',  ( 7.782982007932094604, 15.23835801850285776, 47.04930799450052348 ) ) ;
#25206=DIRECTION ( 'NONE',  ( -0.000000000000000000, -1.000000000000000000, 0.000000000000000000 ) ) ;
#25207=TOROIDAL_SURFACE ( 'NONE', #11055, 41.50000000000000000, 1.499999999999997780 ) ;
#25220=VERTEX_POINT ( 'NONE', #1434 ) ;
#25236=FACE_OUTER_BOUND ( 'NONE', #5005, .T. ) ;
#25238=DIRECTION ( 'NONE',  ( -1.000000000000000000, 0.000000000000000000, 0.000000000000000000 ) ) ;
#25248=DIRECTION ( 'NONE',  ( -1.000000000000000000, 0.000000000000000000, 0.000000000000000000 ) ) ;
#25283=EDGE_CURVE ( 'NONE', #8390, #3586, #4805, .T. ) ;
#25295=AXIS2_PLACEMENT_3D ( 'NONE', #12859, #27784, #364 ) ;
#25314=ORIENTED_EDGE ( 'NONE', *, *, #25664, .F. ) ;
#25337=DIRECTION ( 'NONE',  ( -1.224646799147353207E-16, 0.000000000000000000, -1.000000000000000000 ) ) ;
#25348=CYLINDRICAL_SURFACE ( 'NONE', #7944, 21.50000000000000000 ) ;
#25368=ORIENTED_EDGE ( 'NONE', *, *, #3361, .T. ) ;
#25375=CYLINDRICAL_SURFACE ( 'NONE', #32410, 40.00000000000000711 ) ;
#25385=FACE_OUTER_BOUND ( 'NONE', #4621, .T. ) ;
#25403=EDGE_LOOP ( 'NONE', ( #20762, #15140, #20851, #31318 ) ) ;
#25411=TOROIDAL_SURFACE ( 'NONE', #6008, 32.50000000000000000, 1.499999999999999556 ) ;
#25455=EDGE_CURVE ( 'NONE', #11782, #1013, #13206, .T. ) ;
#25480=ORIENTED_EDGE ( 'NONE', *, *, #30512, .T. ) ;
#25481=DIRECTION ( 'NONE',  ( -0.000000000000000000, -1.000000000000000000, 0.000000000000000000 ) ) ;
#25483=CARTESIAN_POINT ( 'NONE',  ( -24.90080973260340613, 13.80129159329807287, 47.04930799450052348 ) ) ;
#25493=VERTEX_POINT ( 'NONE', #18949 ) ;
#25510=EDGE_LOOP ( 'NONE', ( #5727, #6294, #14717, #826 ) ) ;
#25512=CYLINDRICAL_SURFACE ( 'NONE', #9996, 21.50000000000000000 ) ;
#25514=CARTESIAN_POINT ( 'NONE',  ( 64.09785597605721819, 14.86454579224779948, 47.04930799450051637 ) ) ;
#25535=DIRECTION ( 'NONE',  ( -1.000000000000000000, 0.000000000000000000, 0.000000000000000000 ) ) ;
#25536=AXIS2_PLACEMENT_3D ( 'NONE', #1049, #11075, #18440 ) ;
#25537=ORIENTED_EDGE ( 'NONE', *, *, #5317, .T. ) ;
#25545=ORIENTED_EDGE ( 'NONE', *, *, #30221, .T. ) ;
#25548=ORIENTED_EDGE ( 'NONE', *, *, #29084, .F. ) ;
#25557=CARTESIAN_POINT ( 'NONE',  ( 67.84785597605720397, 13.61454579224779771, 47.04930799450051637 ) ) ;
#25565=ORIENTED_EDGE ( 'NONE', *, *, #27579, .T. ) ;
#25576=FACE_OUTER_BOUND ( 'NONE', #3815, .T. ) ;
#25583=AXIS2_PLACEMENT_3D ( 'NONE', #24066, #9468, #21277 ) ;
#25584=ORIENTED_EDGE ( 'NONE', *, *, #31345, .F. ) ;
#25591=DIRECTION ( 'NONE',  ( 1.000000000000000000, 0.000000000000000000, 0.000000000000000000 ) ) ;
#25595=AXIS2_PLACEMENT_3D ( 'NONE', #13998, #9229, #16446 ) ;
#25596=CARTESIAN_POINT ( 'NONE',  ( 21.09785597605720753, 15.57592086119046826, 47.04930799450052348 ) ) ;
#25598=ORIENTED_EDGE ( 'NONE', *, *, #1815, .F. ) ;
#25601=EDGE_CURVE ( 'NONE', #13599, #17931, #14797, .T. ) ;
#25640=ORIENTED_EDGE ( 'NONE', *, *, #20377, .T. ) ;
#25655=ORIENTED_EDGE ( 'NONE', *, *, #9403, .F. ) ;
#25662=DIRECTION ( 'NONE',  ( -0.000000000000000000, -1.000000000000000000, 0.000000000000000000 ) ) ;
#25664=EDGE_CURVE ( 'NONE', #7765, #18056, #8505, .T. ) ;
#25681=ADVANCED_FACE ( 'NONE', ( #27157 ), #29473, .F. ) ;
#25682=TOROIDAL_SURFACE ( 'NONE', #26185, 44.50000000000000000, 1.499999999999995115 ) ;
#25687=ADVANCED_FACE ( 'NONE', ( #4679 ), #629, .T. ) ;
#25692=AXIS2_PLACEMENT_3D ( 'NONE', #23318, #829, #985 ) ;
#25697=CIRCLE ( 'NONE', #11538, 1.200000000000006617 ) ;
#25701=TOROIDAL_SURFACE ( 'NONE', #23070, 35.50000000000000711, 1.500000000000001332 ) ;
#25709=ORIENTED_EDGE ( 'NONE', *, *, #26065, .F. ) ;
#25716=AXIS2_PLACEMENT_3D ( 'NONE', #2053, #24872, #12075 ) ;
#25732=ORIENTED_EDGE ( 'NONE', *, *, #126, .T. ) ;
#25761=DIRECTION ( 'NONE',  ( -1.224646799147353207E-16, 0.000000000000000000, -1.000000000000000000 ) ) ;
#25771=FACE_OUTER_BOUND ( 'NONE', #21565, .T. ) ;
#25772=DIRECTION ( 'NONE',  ( -1.000000000000000000, 0.000000000000000000, 0.000000000000000000 ) ) ;
#25789=EDGE_LOOP ( 'NONE', ( #10787, #9015, #659, #2217 ) ) ;
#25796=ADVANCED_FACE ( 'NONE', ( #27651 ), #32414, .T. ) ;
#25803=EDGE_CURVE ( 'NONE', #18077, #19861, #18747, .T. ) ;
#25819=EDGE_CURVE ( 'NONE', #31321, #24672, #11431, .T. ) ;
#25824=CARTESIAN_POINT ( 'NONE',  ( 5.864109918520784781, 14.46497581658974063, 47.04930799450052348 ) ) ;
#25847=AXIS2_PLACEMENT_3D ( 'NONE', #16792, #11720, #21381 ) ;
#25849=AXIS2_PLACEMENT_3D ( 'NONE', #3267, #5737, #26399 ) ;
#25852=FACE_OUTER_BOUND ( 'NONE', #11958, .T. ) ;
#25860=CIRCLE ( 'NONE', #8576, 31.50000000000000000 ) ;
#25886=CARTESIAN_POINT ( 'NONE',  ( 21.09785597605720753, 14.98269195386757602, 47.04930799450052348 ) ) ;
#25889=VERTEX_POINT ( 'NONE', #3345 ) ;
#25904=ORIENTED_EDGE ( 'NONE', *, *, #16402, .T. ) ;
#25910=CARTESIAN_POINT ( 'NONE',  ( 21.09785597605720753, 14.86454579224779948, 47.04930799450052348 ) ) ;
#25913=ORIENTED_EDGE ( 'NONE', *, *, #19620, .F. ) ;
#25922=ORIENTED_EDGE ( 'NONE', *, *, #8258, .T. ) ;
#25924=ORIENTED_EDGE ( 'NONE', *, *, #7275, .T. ) ;
#25937=DIRECTION ( 'NONE',  ( -1.000000000000000000, 0.000000000000000000, 0.000000000000000000 ) ) ;
#25938=VERTEX_POINT ( 'NONE', #878 ) ;
#25962=AXIS2_PLACEMENT_3D ( 'NONE', #11575, #23877, #11402 ) ;
#25969=ADVANCED_FACE ( 'NONE', ( #20900 ), #17730, .T. ) ;
#25979=DIRECTION ( 'NONE',  ( -0.9275012328650846793, -0.3738200944756017163, 0.000000000000000000 ) ) ;
#25980=DIRECTION ( 'NONE',  ( -0.000000000000000000, -1.000000000000000000, 0.000000000000000000 ) ) ;
#25992=CARTESIAN_POINT ( 'NONE',  ( -21.90214402394278892, 14.86454579224779948, 47.04930799450052348 ) ) ;
#25997=DIRECTION ( 'NONE',  ( -0.000000000000000000, -1.000000000000000000, 0.000000000000000000 ) ) ;
#26001=ORIENTED_EDGE ( 'NONE', *, *, #28401, .F. ) ;
#26009=DIRECTION ( 'NONE',  ( -1.000000000000000000, 0.000000000000000000, 0.000000000000000000 ) ) ;
#26017=CARTESIAN_POINT ( 'NONE',  ( 21.09785597605720753, 13.61454579224779771, 47.04930799450052348 ) ) ;
#26018=LINE ( 'NONE', #13558, #18900 ) ;
#26041=ORIENTED_EDGE ( 'NONE', *, *, #11524, .F. ) ;
#26050=ORIENTED_EDGE ( 'NONE', *, *, #20038, .F. ) ;
#26052=DIRECTION ( 'NONE',  ( -0.000000000000000000, -1.000000000000000000, 0.000000000000000000 ) ) ;
#26063=LINE ( 'NONE', #16058, #14220 ) ;
#26065=EDGE_CURVE ( 'NONE', #22190, #28560, #419, .T. ) ;
#26069=AXIS2_PLACEMENT_3D ( 'NONE', #1692, #2186, #11712 ) ;
#26091=VERTEX_POINT ( 'NONE', #5460 ) ;
#26093=CARTESIAN_POINT ( 'NONE',  ( 21.09785597605720753, 13.86454579224779948, 47.04930799450052348 ) ) ;
#26126=CIRCLE ( 'NONE', #20351, 15.28675991284684343 ) ;
#26133=EDGE_LOOP ( 'NONE', ( #20169, #25904, #8707, #27241 ) ) ;
#26134=DIRECTION ( 'NONE',  ( -0.000000000000000000, -1.000000000000000000, 0.000000000000000000 ) ) ;
#26138=EDGE_LOOP ( 'NONE', ( #27461, #22935, #6187, #8249 ) ) ;
#26146=DIRECTION ( 'NONE',  ( -0.000000000000000000, -1.000000000000000000, 0.000000000000000000 ) ) ;
#26151=CARTESIAN_POINT ( 'NONE',  ( 21.09785597605720753, 13.86454579224779948, 47.04930799450052348 ) ) ;
#26171=AXIS2_PLACEMENT_3D ( 'NONE', #4410, #11644, #19501 ) ;
#26185=AXIS2_PLACEMENT_3D ( 'NONE', #11737, #21399, #11897 ) ;
#26186=VERTEX_POINT ( 'NONE', #847 ) ;
#26196=VERTEX_POINT ( 'NONE', #26281 ) ;
#26222=CIRCLE ( 'NONE', #2644, 46.27992121592387065 ) ;
#26224=ORIENTED_EDGE ( 'NONE', *, *, #14354, .F. ) ;
#26249=EDGE_CURVE ( 'NONE', #18953, #9681, #10961, .T. ) ;
#26254=AXIS2_PLACEMENT_3D ( 'NONE', #26151, #26478, #23849 ) ;
#26264=FACE_OUTER_BOUND ( 'NONE', #1417, .T. ) ;
#26281=CARTESIAN_POINT ( 'NONE',  ( 34.91272994418231690, 15.57592086119046826, 47.04930799450052348 ) ) ;
#26290=DIRECTION ( 'NONE',  ( -0.000000000000000000, -1.000000000000000000, 0.000000000000000000 ) ) ;
#26299=EDGE_LOOP ( 'NONE', ( #21070, #27232, #15082, #29122 ) ) ;
#26308=DIRECTION ( 'NONE',  ( -0.000000000000000000, -1.000000000000000000, 0.000000000000000000 ) ) ;
#26311=EDGE_LOOP ( 'NONE', ( #31366, #19353, #1595, #19018 ) ) ;
#26318=ORIENTED_EDGE ( 'NONE', *, *, #4413, .T. ) ;
#26319=CIRCLE ( 'NONE', #9576, 33.50000000000000000 ) ;
#26326=DIRECTION ( 'NONE',  ( -0.000000000000000000, -1.000000000000000000, 0.000000000000000000 ) ) ;
#26328=ORIENTED_EDGE ( 'NONE', *, *, #31345, .T. ) ;
#26331=VERTEX_POINT ( 'NONE', #14620 ) ;
#26345=ORIENTED_EDGE ( 'NONE', *, *, #6818, .T. ) ;
#26347=DIRECTION ( 'NONE',  ( -1.224646799147353207E-16, 0.000000000000000000, -1.000000000000000000 ) ) ;
#26352=CARTESIAN_POINT ( 'NONE',  ( 67.63274615763145903, 14.16454579224779842, 47.04930799450051637 ) ) ;
#26353=CARTESIAN_POINT ( 'NONE',  ( -18.90214402394279603, 13.86454579224779948, 47.04930799450052348 ) ) ;
#26381=EDGE_CURVE ( 'NONE', #18056, #15722, #22152, .T. ) ;
#26392=ORIENTED_EDGE ( 'NONE', *, *, #26249, .T. ) ;
#26396=DIRECTION ( 'NONE',  ( -1.000000000000000000, 0.000000000000000000, 0.000000000000000000 ) ) ;
#26399=DIRECTION ( 'NONE',  ( -1.000000000000000000, 0.000000000000000000, 0.000000000000000000 ) ) ;
#26411=AXIS2_PLACEMENT_3D ( 'NONE', #7149, #1566, #31934 ) ;
#26451=ADVANCED_FACE ( 'NONE', ( #166 ), #12658, .F. ) ;
#26476=CARTESIAN_POINT ( 'NONE',  ( 21.09785597605720753, 13.86454579224779948, 47.04930799450052348 ) ) ;
#26478=DIRECTION ( 'NONE',  ( -0.000000000000000000, -1.000000000000000000, 0.000000000000000000 ) ) ;
#26482=DIRECTION ( 'NONE',  ( -0.000000000000000000, -1.000000000000000000, 0.000000000000000000 ) ) ;
#26485=CARTESIAN_POINT ( 'NONE',  ( 21.09785597605720753, 14.99513937955032716, 47.04930799450052348 ) ) ;
#26490=FACE_OUTER_BOUND ( 'NONE', #9889, .T. ) ;
#26504=ORIENTED_EDGE ( 'NONE', *, *, #25455, .F. ) ;
#26510=CARTESIAN_POINT ( 'NONE',  ( -24.83466114100572852, 14.61319044934410627, 47.04930799450052348 ) ) ;
#26513=CARTESIAN_POINT ( 'NONE',  ( 21.09785597605720753, 17.16474120167318063, 47.04930799450052348 ) ) ;
#26522=CARTESIAN_POINT ( 'NONE',  ( 50.59785597605720397, 14.86454579224779948, 47.04930799450051637 ) ) ;
#26525=ORIENTED_EDGE ( 'NONE', *, *, #8803, .F. ) ;
#26527=CIRCLE ( 'NONE', #21803, 13.50178401536290984 ) ;
#26535=ORIENTED_EDGE ( 'NONE', *, *, #1296, .F. ) ;
#26540=DIRECTION ( 'NONE',  ( -0.000000000000000000, -1.000000000000000000, 0.000000000000000000 ) ) ;
#26545=VERTEX_POINT ( 'NONE', #12491 ) ;
#26548=EDGE_LOOP ( 'NONE', ( #25922, #7037, #28188, #11770 ) ) ;
#26552=DIRECTION ( 'NONE',  ( -1.000000000000000000, 0.000000000000000000, 0.000000000000000000 ) ) ;
#26553=CARTESIAN_POINT ( 'NONE',  ( -18.40214402394278892, 13.86454579224779948, 47.04930799450052348 ) ) ;
#26565=CARTESIAN_POINT ( 'NONE',  ( -25.57662701300441555, 13.66454579224780019, 47.04930799450052348 ) ) ;
#26575=DIRECTION ( 'NONE',  ( -0.000000000000000000, -1.000000000000000000, 0.000000000000000000 ) ) ;
#26576=LINE ( 'NONE', #4086, #17611 ) ;
#26593=EDGE_CURVE ( 'NONE', #8390, #14305, #7294, .T. ) ;
#26611=CIRCLE ( 'NONE', #29237, 39.49999999999999289 ) ;
#26625=FACE_OUTER_BOUND ( 'NONE', #15055, .T. ) ;
#26639=DIRECTION ( 'NONE',  ( -0.000000000000000000, -1.000000000000000000, 0.000000000000000000 ) ) ;
#26660=AXIS2_PLACEMENT_3D ( 'NONE', #6258, #31053, #6420 ) ;
#26662=EDGE_LOOP ( 'NONE', ( #19889, #16118, #32316, #28771 ) ) ;
#26663=CYLINDRICAL_SURFACE ( 'NONE', #2601, 31.50000000000000000 ) ;
#26690=AXIS2_PLACEMENT_3D ( 'NONE', #25596, #13139, #15748 ) ;
#26691=EDGE_LOOP ( 'NONE', ( #18666, #10885, #2986, #24960 ) ) ;
#26692=EDGE_CURVE ( 'NONE', #18982, #7619, #3013, .T. ) ;
#26720=CARTESIAN_POINT ( 'NONE',  ( 21.09785597605720753, 13.86454579224779948, 47.04930799450052348 ) ) ;
#26722=DIRECTION ( 'NONE',  ( 0.000000000000000000, 0.000000000000000000, 1.000000000000000000 ) ) ;
#26729=LINE ( 'NONE', #9175, #3556 ) ;
#26735=EDGE_LOOP ( 'NONE', ( #25598, #5872, #7766, #29723 ) ) ;
#26775=AXIS2_PLACEMENT_3D ( 'NONE', #16532, #2088, #12116 ) ;
#26782=AXIS2_PLACEMENT_3D ( 'NONE', #29843, #2752, #8008 ) ;
#26832=DIRECTION ( 'NONE',  ( -1.000000000000000000, 0.000000000000000000, 0.000000000000000000 ) ) ;
#26838=DIRECTION ( 'NONE',  ( -0.000000000000000000, -1.000000000000000000, 0.000000000000000000 ) ) ;
#26839=CARTESIAN_POINT ( 'NONE',  ( 40.59785597605721108, 13.86454579224779948, 47.04930799450052348 ) ) ;
#26852=EDGE_LOOP ( 'NONE', ( #12143, #5940, #1856, #6240 ) ) ;
#26863=EDGE_LOOP ( 'NONE', ( #25709, #19789, #18349, #25089 ) ) ;
#26886=DIRECTION ( 'NONE',  ( -0.000000000000000000, -1.000000000000000000, 0.000000000000000000 ) ) ;
#26892=CARTESIAN_POINT ( 'NONE',  ( 21.09785597605720753, 15.57592086119046826, 47.04930799450052348 ) ) ;
#26896=DIRECTION ( 'NONE',  ( -1.000000000000000000, 0.000000000000000000, 0.000000000000000000 ) ) ;
#26910=ORIENTED_EDGE ( 'NONE', *, *, #30629, .T. ) ;
#26916=ORIENTED_EDGE ( 'NONE', *, *, #1296, .T. ) ;
#26936=VECTOR ( 'NONE', #4846, 1000.000000000000000 ) ;
#26938=ORIENTED_EDGE ( 'NONE', *, *, #9543, .F. ) ;
#26940=CARTESIAN_POINT ( 'NONE',  ( -16.40214402394279958, 14.86454579224779948, 47.04930799450052348 ) ) ;
#26944=ORIENTED_EDGE ( 'NONE', *, *, #22205, .T. ) ;
#26963=DIRECTION ( 'NONE',  ( -1.000000000000000000, 0.000000000000000000, 0.000000000000000000 ) ) ;
#26977=ORIENTED_EDGE ( 'NONE', *, *, #9122, .T. ) ;
#27004=CYLINDRICAL_SURFACE ( 'NONE', #27306, 43.00000000000000000 ) ;
#27009=DIRECTION ( 'NONE',  ( -0.000000000000000000, -1.000000000000000000, 0.000000000000000000 ) ) ;
#27017=( GEOMETRIC_REPRESENTATION_CONTEXT ( 3 ) GLOBAL_UNCERTAINTY_ASSIGNED_CONTEXT ( ( #10811 ) ) GLOBAL_UNIT_ASSIGNED_CONTEXT ( ( #14172, #32051, #29252 ) ) REPRESENTATION_CONTEXT ( 'NONE', 'WORKASPACE' ) );
#27019=ORIENTED_EDGE ( 'NONE', *, *, #16737, .T. ) ;
#27029=CARTESIAN_POINT ( 'NONE',  ( 21.09785597605720753, 13.86454579224779948, 47.04930799450052348 ) ) ;
#27052=LINE ( 'NONE', #2272, #5902 ) ;
#27059=VERTEX_POINT ( 'NONE', #16306 ) ;
#27062=CARTESIAN_POINT ( 'NONE',  ( 21.09785597605720753, 17.16474120167318418, 47.04930799450052348 ) ) ;
#27070=ORIENTED_EDGE ( 'NONE', *, *, #23066, .T. ) ;
#27072=ORIENTED_EDGE ( 'NONE', *, *, #17675, .F. ) ;
#27090=ORIENTED_EDGE ( 'NONE', *, *, #8252, .F. ) ;
#27101=CARTESIAN_POINT ( 'NONE',  ( 0.5978559760572086379, 13.86454579224779948, 47.04930799450052348 ) ) ;
#27109=EDGE_CURVE ( 'NONE', #21091, #1796, #5760, .T. ) ;
#27143=CARTESIAN_POINT ( 'NONE',  ( 21.09785597605720753, 15.57592086119046826, 47.04930799450052348 ) ) ;
#27145=CONICAL_SURFACE ( 'NONE', #11952, 13.81487396812510937, 1.187672012580059944 ) ;
#27148=DIRECTION ( 'NONE',  ( -1.000000000000000000, 0.000000000000000000, 0.000000000000000000 ) ) ;
#27152=CARTESIAN_POINT ( 'NONE',  ( -3.902144023942792028, 13.86454579224779948, 47.04930799450052348 ) ) ;
#27155=DIRECTION ( 'NONE',  ( 1.000000000000000000, 0.000000000000000000, 0.000000000000000000 ) ) ;
#27157=FACE_OUTER_BOUND ( 'NONE', #15345, .T. ) ;
#27166=ORIENTED_EDGE ( 'NONE', *, *, #16737, .F. ) ;
#27168=ORIENTED_EDGE ( 'NONE', *, *, #13286, .F. ) ;
#27169=ORIENTED_EDGE ( 'NONE', *, *, #8490, .F. ) ;
#27185=ORIENTED_EDGE ( 'NONE', *, *, #21993, .T. ) ;
#27186=CARTESIAN_POINT ( 'NONE',  ( 21.09785597605720753, 13.86454579224779948, 47.04930799450052348 ) ) ;
#27225=DIRECTION ( 'NONE',  ( -0.000000000000000000, -1.000000000000000000, 0.000000000000000000 ) ) ;
#27232=ORIENTED_EDGE ( 'NONE', *, *, #31273, .T. ) ;
#27241=ORIENTED_EDGE ( 'NONE', *, *, #710, .F. ) ;
#27250=DIRECTION ( 'NONE',  ( -1.000000000000000000, 0.000000000000000000, 0.000000000000000000 ) ) ;
#27252=VECTOR ( 'NONE', #9906, 1000.000000000000000 ) ;
#27254=AXIS2_PLACEMENT_3D ( 'NONE', #22719, #25662, #2851 ) ;
#27259=ORIENTED_EDGE ( 'NONE', *, *, #5754, .F. ) ;
#27263=DIRECTION ( 'NONE',  ( -1.000000000000000000, 0.000000000000000000, 0.000000000000000000 ) ) ;
#27269=ADVANCED_FACE ( 'NONE', ( #22204 ), #9464, .T. ) ;
#27274=DIRECTION ( 'NONE',  ( -1.000000000000000000, 0.000000000000000000, 0.000000000000000000 ) ) ;
#27276=DIRECTION ( 'NONE',  ( -0.000000000000000000, -1.000000000000000000, 0.000000000000000000 ) ) ;
#27284=EDGE_LOOP ( 'NONE', ( #431, #25640, #32011, #4692 ) ) ;
#27287=DIRECTION ( 'NONE',  ( -1.000000000000000000, 0.000000000000000000, 0.000000000000000000 ) ) ;
#27306=AXIS2_PLACEMENT_3D ( 'NONE', #29965, #19767, #16819 ) ;
#27313=AXIS2_PLACEMENT_3D ( 'NONE', #24537, #2055, #12077 ) ;
#27317=DIRECTION ( 'NONE',  ( -1.000000000000000000, 0.000000000000000000, 0.000000000000000000 ) ) ;
#27320=ORIENTED_EDGE ( 'NONE', *, *, #3110, .T. ) ;
#27346=ORIENTED_EDGE ( 'NONE', *, *, #18868, .T. ) ;
#27349=EDGE_CURVE ( 'NONE', #29185, #15519, #26222, .T. ) ;
#27363=DIRECTION ( 'NONE',  ( -1.000000000000000000, 0.000000000000000000, 0.000000000000000000 ) ) ;
#27378=DIRECTION ( 'NONE',  ( -0.000000000000000000, -1.000000000000000000, 0.000000000000000000 ) ) ;
#27416=DIRECTION ( 'NONE',  ( -1.000000000000000000, 0.000000000000000000, 0.000000000000000000 ) ) ;
#27461=ORIENTED_EDGE ( 'NONE', *, *, #31668, .T. ) ;
#27476=EDGE_CURVE ( 'NONE', #19635, #9965, #30743, .T. ) ;
#27481=VERTEX_POINT ( 'NONE', #5141 ) ;
#27490=AXIS2_PLACEMENT_3D ( 'NONE', #6161, #21246, #13406 ) ;
#27514=AXIS2_PLACEMENT_3D ( 'NONE', #17832, #7174, #27363 ) ;
#27518=ORIENTED_EDGE ( 'NONE', *, *, #20041, .T. ) ;
#27530=DIRECTION ( 'NONE',  ( -0.000000000000000000, -1.000000000000000000, 0.000000000000000000 ) ) ;
#27538=DIRECTION ( 'NONE',  ( -1.000000000000000000, 0.000000000000000000, 0.000000000000000000 ) ) ;
#27560=CARTESIAN_POINT ( 'NONE',  ( 21.09785597605720753, -5.098646251524523443, 47.04930799450052348 ) ) ;
#27569=DIRECTION ( 'NONE',  ( -0.000000000000000000, -1.000000000000000000, 0.000000000000000000 ) ) ;
#27572=DIRECTION ( 'NONE',  ( -0.000000000000000000, -1.000000000000000000, 0.000000000000000000 ) ) ;
#27573=FACE_OUTER_BOUND ( 'NONE', #10748, .T. ) ;
#27579=EDGE_CURVE ( 'NONE', #665, #17919, #25697, .T. ) ;
#27651=FACE_OUTER_BOUND ( 'NONE', #26852, .T. ) ;
#27656=DIRECTION ( 'NONE',  ( 0.000000000000000000, 0.000000000000000000, 1.000000000000000000 ) ) ;
#27668=EDGE_CURVE ( 'NONE', #663, #18077, #2316, .T. ) ;
#27672=FACE_OUTER_BOUND ( 'NONE', #764, .T. ) ;
#27675=EDGE_CURVE ( 'NONE', #11329, #6385, #19869, .T. ) ;
#27687=DIRECTION ( 'NONE',  ( 0.000000000000000000, 0.000000000000000000, 1.000000000000000000 ) ) ;
#27698=EDGE_CURVE ( 'NONE', #7100, #9965, #4746, .T. ) ;
#27699=CARTESIAN_POINT ( 'NONE',  ( 34.91272994418231690, 15.57592086119046826, 47.04930799450052348 ) ) ;
#27704=CARTESIAN_POINT ( 'NONE',  ( 21.09785597605720753, 13.86454579224779948, 47.04930799450052348 ) ) ;
#27716=CIRCLE ( 'NONE', #18287, 21.50000000000000000 ) ;
#27726=ORIENTED_EDGE ( 'NONE', *, *, #22973, .T. ) ;
#27751=ORIENTED_EDGE ( 'NONE', *, *, #15247, .T. ) ;
#27772=( LENGTH_UNIT ( ) NAMED_UNIT ( * ) SI_UNIT ( .MILLI., .METRE. ) );
#27784=DIRECTION ( 'NONE',  ( -0.000000000000000000, -1.000000000000000000, 0.000000000000000000 ) ) ;
#27797=CARTESIAN_POINT ( 'NONE',  ( 56.59785597605721108, 14.86454579224779948, 47.04930799450051637 ) ) ;
#27817=DIRECTION ( 'NONE',  ( -1.000000000000000000, 0.000000000000000000, 0.000000000000000000 ) ) ;
#27835=AXIS2_PLACEMENT_3D ( 'NONE', #17677, #19809, #27538 ) ;
#27844=EDGE_LOOP ( 'NONE', ( #14711, #22075, #22881, #32377 ) ) ;
#27852=ORIENTED_EDGE ( 'NONE', *, *, #20291, .F. ) ;
#27861=DIRECTION ( 'NONE',  ( -0.000000000000000000, -1.000000000000000000, 0.000000000000000000 ) ) ;
#27869=ORIENTED_EDGE ( 'NONE', *, *, #10614, .T. ) ;
#27875=EDGE_LOOP ( 'NONE', ( #5645, #27726, #1902, #15393 ) ) ;
#27886=ADVANCED_FACE ( 'NONE', ( #30057 ), #22652, .T. ) ;
#27924=DIRECTION ( 'NONE',  ( -1.000000000000000000, 0.000000000000000000, 0.000000000000000000 ) ) ;
#27926=CARTESIAN_POINT ( 'NONE',  ( 34.09963999142011204, -5.098646251524523443, 47.04930799450052348 ) ) ;
#27939=ORIENTED_EDGE ( 'NONE', *, *, #18617, .T. ) ;
#27946=DIRECTION ( 'NONE',  ( -0.000000000000000000, -1.000000000000000000, 0.000000000000000000 ) ) ;
#27954=ADVANCED_FACE ( 'NONE', ( #11319 ), #28394, .T. ) ;
#27959=TOROIDAL_SURFACE ( 'NONE', #15889, 41.50000000000000000, 1.499999999999997780 ) ;
#27960=DIRECTION ( 'NONE',  ( -0.000000000000000000, -1.000000000000000000, 0.000000000000000000 ) ) ;
#27961=FACE_OUTER_BOUND ( 'NONE', #12939, .T. ) ;
#27966=TOROIDAL_SURFACE ( 'NONE', #25849, 46.53489018157424084, 0.7000000000000002887 ) ;
#27979=CARTESIAN_POINT ( 'NONE',  ( 7.596071960694297687, 15.70210863493540288, 47.04930799450052348 ) ) ;
#28030=EDGE_CURVE ( 'NONE', #2441, #13945, #24606, .T. ) ;
#28032=AXIS2_PLACEMENT_3D ( 'NONE', #10366, #11015, #18064 ) ;
#28054=CIRCLE ( 'NONE', #15475, 37.00000000000000711 ) ;
#28057=CIRCLE ( 'NONE', #801, 37.00000000000000711 ) ;
#28061=FACE_OUTER_BOUND ( 'NONE', #23850, .T. ) ;
#28063=FACE_OUTER_BOUND ( 'NONE', #3041, .T. ) ;
#28069=DIRECTION ( 'NONE',  ( -1.000000000000000000, 0.000000000000000000, 0.000000000000000000 ) ) ;
#28074=EDGE_CURVE ( 'NONE', #665, #31921, #7852, .T. ) ;
#28079=TOROIDAL_SURFACE ( 'NONE', #23869, 23.50000000000000000, 2.000000000000001776 ) ;
#28081=AXIS2_PLACEMENT_3D ( 'NONE', #9437, #6970, #1387 ) ;
#28097=DIRECTION ( 'NONE',  ( -1.000000000000000000, 0.000000000000000000, 0.000000000000000000 ) ) ;
#28098=EDGE_CURVE ( 'NONE', #25493, #9681, #28802, .T. ) ;
#28127=DIRECTION ( 'NONE',  ( -0.000000000000000000, -1.000000000000000000, 0.000000000000000000 ) ) ;
#28133=ADVANCED_FACE ( 'NONE', ( #9504 ), #31948, .T. ) ;
#28139=CARTESIAN_POINT ( 'NONE',  ( 41.59785597605720397, 13.86454579224779948, 47.04930799450052348 ) ) ;
#28146=DIRECTION ( 'NONE',  ( -0.000000000000000000, -1.000000000000000000, 0.000000000000000000 ) ) ;
#28147=CARTESIAN_POINT ( 'NONE',  ( 21.09785597605720753, 13.86454579224779948, 47.04930799450052348 ) ) ;
#28152=CARTESIAN_POINT ( 'NONE',  ( 21.09785597605720753, 14.61319044934410627, 47.04930799450052348 ) ) ;
#28157=ORIENTED_EDGE ( 'NONE', *, *, #11434, .T. ) ;
#28167=ORIENTED_EDGE ( 'NONE', *, *, #27668, .T. ) ;
#28180=ORIENTED_EDGE ( 'NONE', *, *, #24442, .F. ) ;
#28188=ORIENTED_EDGE ( 'NONE', *, *, #32281, .F. ) ;
#28227=DIRECTION ( 'NONE',  ( -1.000000000000000000, 0.000000000000000000, 0.000000000000000000 ) ) ;
#28254=DIRECTION ( 'NONE',  ( -1.000000000000000000, 0.000000000000000000, 0.000000000000000000 ) ) ;
#28264=CIRCLE ( 'NONE', #14110, 0.5000000000000004441 ) ;
#28271=DIRECTION ( 'NONE',  ( -1.000000000000000000, 0.000000000000000000, 0.000000000000000000 ) ) ;
#28301=DIRECTION ( 'NONE',  ( -1.000000000000000000, 0.000000000000000000, 0.000000000000000000 ) ) ;
#28309=ADVANCED_FACE ( 'NONE', ( #4902 ), #11005, .T. ) ;
#28343=AXIS2_PLACEMENT_3D ( 'NONE', #10021, #12485, #25591 ) ;
#28347=CARTESIAN_POINT ( 'NONE',  ( 75.19785597605721250, 14.56454579224780055, 47.04930799450051637 ) ) ;
#28379=AXIS2_PLACEMENT_3D ( 'NONE', #22346, #30397, #10215 ) ;
#28390=CARTESIAN_POINT ( 'NONE',  ( 68.16890023319646730, 14.86454579224779948, 47.04930799450052348 ) ) ;
#28394=CYLINDRICAL_SURFACE ( 'NONE', #11562, 40.00000000000000711 ) ;
#28401=EDGE_CURVE ( 'NONE', #30896, #15810, #5786, .T. ) ;
#28402=EDGE_CURVE ( 'NONE', #17364, #5196, #14167, .T. ) ;
#28405=ORIENTED_EDGE ( 'NONE', *, *, #31390, .F. ) ;
#28408=CYLINDRICAL_SURFACE ( 'NONE', #17289, 43.00000000000000000 ) ;
#28441=EDGE_CURVE ( 'NONE', #31321, #18804, #17292, .T. ) ;
#28468=ORIENTED_EDGE ( 'NONE', *, *, #14026, .T. ) ;
#28480=AXIS2_PLACEMENT_3D ( 'NONE', #25057, #17004, #10131 ) ;
#28484=CIRCLE ( 'NONE', #21644, 0.2000000000000057288 ) ;
#28486=FACE_OUTER_BOUND ( 'NONE', #17466, .T. ) ;
#28488=DIRECTION ( 'NONE',  ( -0.000000000000000000, -1.000000000000000000, 0.000000000000000000 ) ) ;
#28491=FACE_OUTER_BOUND ( 'NONE', #12505, .T. ) ;
#28501=LINE ( 'NONE', #31605, #22078 ) ;
#28529=ADVANCED_FACE ( 'NONE', ( #10896 ), #16235, .F. ) ;
#28549=FACE_OUTER_BOUND ( 'NONE', #2439, .T. ) ;
#28560=VERTEX_POINT ( 'NONE', #21047 ) ;
#28561=VECTOR ( 'NONE', #6570, 1000.000000000000000 ) ;
#28562=EDGE_LOOP ( 'NONE', ( #26041, #16352, #14525, #23037 ) ) ;
#28571=DIRECTION ( 'NONE',  ( -0.000000000000000000, -1.000000000000000000, 0.000000000000000000 ) ) ;
#28574=EDGE_CURVE ( 'NONE', #294, #26091, #16, .T. ) ;
#28583=DIRECTION ( 'NONE',  ( -1.000000000000000000, 0.000000000000000000, 0.000000000000000000 ) ) ;
#28604=ORIENTED_EDGE ( 'NONE', *, *, #3982, .F. ) ;
#28618=DIRECTION ( 'NONE',  ( -1.000000000000000000, 0.000000000000000000, 0.000000000000000000 ) ) ;
#28621=DIRECTION ( 'NONE',  ( -0.000000000000000000, -1.000000000000000000, 0.000000000000000000 ) ) ;
#28622=VERTEX_POINT ( 'NONE', #30727 ) ;
#28643=CARTESIAN_POINT ( 'NONE',  ( 21.09785597605720753, -5.098646251524523443, 47.04930799450052348 ) ) ;
#28655=ORIENTED_EDGE ( 'NONE', *, *, #5461, .F. ) ;
#28663=DIRECTION ( 'NONE',  ( 1.000000000000000000, 0.000000000000000000, 0.000000000000000000 ) ) ;
#28664=EDGE_LOOP ( 'NONE', ( #28809, #27751, #10292, #26938 ) ) ;
#28671=ADVANCED_FACE ( 'NONE', ( #22838 ), #15457, .F. ) ;
#28674=AXIS2_PLACEMENT_3D ( 'NONE', #5983, #13696, #28780 ) ;
#28684=EDGE_CURVE ( 'NONE', #7619, #17055, #23585, .T. ) ;
#28696=DIRECTION ( 'NONE',  ( -1.000000000000000000, 0.000000000000000000, 0.000000000000000000 ) ) ;
#28708=CARTESIAN_POINT ( 'NONE',  ( 21.09785597605720753, -5.098646251524523443, 47.04930799450052348 ) ) ;
#28721=ORIENTED_EDGE ( 'NONE', *, *, #2840, .F. ) ;
#28748=CIRCLE ( 'NONE', #14600, 2.000000000000001776 ) ;
#28771=ORIENTED_EDGE ( 'NONE', *, *, #9626, .T. ) ;
#28778=DIRECTION ( 'NONE',  ( -0.000000000000000000, -1.000000000000000000, 0.000000000000000000 ) ) ;
#28780=DIRECTION ( 'NONE',  ( -1.000000000000000000, 0.000000000000000000, 0.000000000000000000 ) ) ;
#28792=AXIS2_PLACEMENT_3D ( 'NONE', #18756, #19737, #14344 ) ;
#28800=AXIS2_PLACEMENT_3D ( 'NONE', #212, #29761, #2353 ) ;
#28802=CIRCLE ( 'NONE', #16749, 0.7000000000000061728 ) ;
#28809=ORIENTED_EDGE ( 'NONE', *, *, #19783, .F. ) ;
#28810=DIRECTION ( 'NONE',  ( -0.000000000000000000, -1.000000000000000000, 0.000000000000000000 ) ) ;
#28814=ORIENTED_EDGE ( 'NONE', *, *, #20892, .T. ) ;
#28816=DIRECTION ( 'NONE',  ( -0.000000000000000000, -1.000000000000000000, 0.000000000000000000 ) ) ;
#28820=EDGE_LOOP ( 'NONE', ( #16883, #5304, #14991, #11966 ) ) ;
#28899=ORIENTED_EDGE ( 'NONE', *, *, #20642, .F. ) ;
#28950=ORIENTED_EDGE ( 'NONE', *, *, #3259, .F. ) ;
#28954=FACE_OUTER_BOUND ( 'NONE', #6556, .T. ) ;
#28964=CIRCLE ( 'NONE', #29484, 2.000000000000001776 ) ;
#29008=AXIS2_PLACEMENT_3D ( 'NONE', #21837, #6267, #16272 ) ;
#29021=EDGE_CURVE ( 'NONE', #1158, #9965, #31475, .T. ) ;
#29035=DIRECTION ( 'NONE',  ( 0.000000000000000000, 0.000000000000000000, 1.000000000000000000 ) ) ;
#29042=DIRECTION ( 'NONE',  ( -1.224646799147353207E-16, 0.000000000000000000, -1.000000000000000000 ) ) ;
#29045=LINE ( 'NONE', #6719, #19391 ) ;
#29049=DIRECTION ( 'NONE',  ( -1.000000000000000000, 0.000000000000000000, 0.000000000000000000 ) ) ;
#29055=AXIS2_PLACEMENT_3D ( 'NONE', #8221, #8700, #13474 ) ;
#29062=CARTESIAN_POINT ( 'NONE',  ( 21.09785597605720753, 17.16474120167318063, 47.04930799450052348 ) ) ;
#29071=AXIS2_PLACEMENT_3D ( 'NONE', #31039, #15290, #13479 ) ;
#29072=ADVANCED_FACE ( 'NONE', ( #28063 ), #25207, .F. ) ;
#29084=EDGE_CURVE ( 'NONE', #4784, #29883, #5293, .T. ) ;
#29097=ADVANCED_FACE ( 'NONE', ( #17392 ), #23629, .F. ) ;
#29118=DIRECTION ( 'NONE',  ( -0.000000000000000000, -1.000000000000000000, 0.000000000000000000 ) ) ;
#29122=ORIENTED_EDGE ( 'NONE', *, *, #2834, .F. ) ;
#29125=MECHANICAL_DESIGN_GEOMETRIC_PRESENTATION_REPRESENTATION('',(#12885),#20732);
#29126=EDGE_CURVE ( 'NONE', #8390, #13490, #26063, .T. ) ;
#29128=EDGE_CURVE ( 'NONE', #19572, #19635, #20483, .T. ) ;
#29164=PRODUCT_DEFINITION_FORMATION_WITH_SPECIFIED_SOURCE ( 'ANY', '', #29749, .NOT_KNOWN. ) ;
#29180=CARTESIAN_POINT ( 'NONE',  ( 48.59785597605719687, 13.86454579224779948, 47.04930799450052348 ) ) ;
#29184=DIRECTION ( 'NONE',  ( -1.000000000000000000, 0.000000000000000000, 0.000000000000000000 ) ) ;
#29185=VERTEX_POINT ( 'NONE', #8203 ) ;
#29200=ADVANCED_FACE ( 'NONE', ( #20823 ), #15779, .F. ) ;
#29213=AXIS2_PLACEMENT_3D ( 'NONE', #20549, #25481, #30095 ) ;
#29221=ORIENTED_EDGE ( 'NONE', *, *, #24913, .T. ) ;
#29237=AXIS2_PLACEMENT_3D ( 'NONE', #31495, #16697, #18998 ) ;
#29241=CIRCLE ( 'NONE', #31342, 1.500000000000001332 ) ;
#29247=FACE_OUTER_BOUND ( 'NONE', #861, .T. ) ;
#29252=( NAMED_UNIT ( * ) SI_UNIT ( $, .STERADIAN. ) SOLID_ANGLE_UNIT ( ) );
#29292=DIRECTION ( 'NONE',  ( -1.000000000000000000, 0.000000000000000000, 0.000000000000000000 ) ) ;
#29324=CARTESIAN_POINT ( 'NONE',  ( 21.09785597605720753, -5.098646251524523443, 47.04930799450052348 ) ) ;
#29331=FACE_OUTER_BOUND ( 'NONE', #27844, .T. ) ;
#29338=AXIS2_PLACEMENT_3D ( 'NONE', #16308, #26326, #29607 ) ;
#29340=DIRECTION ( 'NONE',  ( -1.000000000000000000, 0.000000000000000000, 0.000000000000000000 ) ) ;
#29351=ADVANCED_FACE ( 'NONE', ( #127 ), #4253, .F. ) ;
#29371=CIRCLE ( 'NONE', #16271, 21.49999999999999645 ) ;
#29373=FACE_OUTER_BOUND ( 'NONE', #30136, .T. ) ;
#29386=ORIENTED_EDGE ( 'NONE', *, *, #30629, .F. ) ;
#29393=EDGE_CURVE ( 'NONE', #13364, #10403, #13676, .T. ) ;
#29406=AXIS2_PLACEMENT_3D ( 'NONE', #30565, #30726, #20859 ) ;
#29419=TOROIDAL_SURFACE ( 'NONE', #26254, 26.49999999999999645, 1.499999999999997780 ) ;
#29431=DIRECTION ( 'NONE',  ( -0.000000000000000000, -1.000000000000000000, 0.000000000000000000 ) ) ;
#29439=ORIENTED_EDGE ( 'NONE', *, *, #26593, .F. ) ;
#29444=CARTESIAN_POINT ( 'NONE',  ( 64.09785597605721819, 13.86454579224779948, 47.04930799450051637 ) ) ;
#29473=CYLINDRICAL_SURFACE ( 'NONE', #3248, 25.00000000000000000 ) ;
#29477=CYLINDRICAL_SURFACE ( 'NONE', #12680, 37.50000000000000711 ) ;
#29479=ORIENTED_EDGE ( 'NONE', *, *, #22250, .T. ) ;
#29484=AXIS2_PLACEMENT_3D ( 'NONE', #20696, #20858, #11023 ) ;
#29491=EDGE_CURVE ( 'NONE', #18936, #17919, #23650, .T. ) ;
#29493=EDGE_CURVE ( 'NONE', #15722, #1158, #9506, .T. ) ;
#29501=CIRCLE ( 'NONE', #8555, 1.290569415042096324 ) ;
#29515=CARTESIAN_POINT ( 'NONE',  ( 47.59785597605720397, 13.86454579224779948, 47.04930799450052348 ) ) ;
#29517=AXIS2_PLACEMENT_3D ( 'NONE', #6030, #18643, #23265 ) ;
#29535=TOROIDAL_SURFACE ( 'NONE', #15387, 20.49999999999999645, 1.499999999999997780 ) ;
#29536=AXIS2_PLACEMENT_3D ( 'NONE', #14577, #19321, #29184 ) ;
#29547=EDGE_LOOP ( 'NONE', ( #8673, #2827, #25368, #19829 ) ) ;
#29554=AXIS2_PLACEMENT_3D ( 'NONE', #8319, #15701, #8165 ) ;
#29571=ORIENTED_EDGE ( 'NONE', *, *, #18617, .F. ) ;
#29600=EDGE_LOOP ( 'NONE', ( #24230, #20090 ) ) ;
#29607=DIRECTION ( 'NONE',  ( -1.000000000000000000, 0.000000000000000000, 0.000000000000000000 ) ) ;
#29608=DIRECTION ( 'NONE',  ( -1.000000000000000000, 0.000000000000000000, 0.000000000000000000 ) ) ;
#29631=EDGE_LOOP ( 'NONE', ( #25548, #22369, #30100, #23352 ) ) ;
#29632=DIRECTION ( 'NONE',  ( 0.000000000000000000, 0.000000000000000000, 1.000000000000000000 ) ) ;
#29635=CARTESIAN_POINT ( 'NONE',  ( 21.09785597605720753, -5.098646251524523443, 47.04930799450052348 ) ) ;
#29640=CARTESIAN_POINT ( 'NONE',  ( 38.59785597605721108, 14.86454579224779948, 47.04930799450052348 ) ) ;
#29650=COLOUR_RGB ( '',0.7921568627450980005, 0.8196078431372548767, 0.9333333333333333481 ) ;
#29656=ADVANCED_FACE ( 'NONE', ( #18954 ), #29477, .T. ) ;
#29657=ORIENTED_EDGE ( 'NONE', *, *, #17980, .T. ) ;
#29658=ORIENTED_EDGE ( 'NONE', *, *, #4346, .F. ) ;
#29662=FACE_OUTER_BOUND ( 'NONE', #5566, .T. ) ;
#29680=EDGE_CURVE ( 'NONE', #3586, #18233, #19464, .T. ) ;
#29698=EDGE_CURVE ( 'NONE', #23541, #5196, #10048, .T. ) ;
#29712=CARTESIAN_POINT ( 'NONE',  ( -3.902144023942795581, -5.098646251524523443, 47.04930799450052348 ) ) ;
#29722=CARTESIAN_POINT ( 'NONE',  ( 7.796202261960367252, 17.36474115922713324, 47.04930799450052348 ) ) ;
#29723=ORIENTED_EDGE ( 'NONE', *, *, #18868, .F. ) ;
#29728=CARTESIAN_POINT ( 'NONE',  ( 21.09785597605720753, 13.95840365082257151, 47.04930799450052348 ) ) ;
#29739=VERTEX_POINT ( 'NONE', #247 ) ;
#29749=PRODUCT ( 'Lower Suspension', 'Lower Suspension', '', ( #7714 ) ) ;
#29756=LINE ( 'NONE', #19230, #402 ) ;
#29760=FACE_OUTER_BOUND ( 'NONE', #22100, .T. ) ;
#29761=DIRECTION ( 'NONE',  ( -0.000000000000000000, -1.000000000000000000, 0.000000000000000000 ) ) ;
#29768=EDGE_CURVE ( 'NONE', #18804, #23918, #32073, .T. ) ;
#29770=EDGE_CURVE ( 'NONE', #15058, #12822, #4789, .T. ) ;
#29774=AXIS2_PLACEMENT_3D ( 'NONE', #16634, #21563, #6643 ) ;
#29777=EDGE_LOOP ( 'NONE', ( #2564, #18700, #8781, #6360 ) ) ;
#29779=DIRECTION ( 'NONE',  ( -1.000000000000000000, 0.000000000000000000, 0.000000000000000000 ) ) ;
#29786=AXIS2_PLACEMENT_3D ( 'NONE', #27979, #243, #15655 ) ;
#29801=CARTESIAN_POINT ( 'NONE',  ( 21.09785597605720753, 14.86454579224779948, 47.04930799450052348 ) ) ;
#29805=EDGE_CURVE ( 'NONE', #17230, #4784, #15289, .T. ) ;
#29817=AXIS2_PLACEMENT_3D ( 'NONE', #5258, #20184, #10513 ) ;
#29843=CARTESIAN_POINT ( 'NONE',  ( 21.09785597605720753, 14.86454579224779948, 47.04930799450052348 ) ) ;
#29850=DIRECTION ( 'NONE',  ( -1.000000000000000000, 0.000000000000000000, 0.000000000000000000 ) ) ;
#29883=VERTEX_POINT ( 'NONE', #25992 ) ;
#29901=EDGE_LOOP ( 'NONE', ( #27090, #24937, #6585, #21333 ) ) ;
#29902=ORIENTED_EDGE ( 'NONE', *, *, #31668, .F. ) ;
#29904=FACE_OUTER_BOUND ( 'NONE', #11206, .T. ) ;
#29946=DIRECTION ( 'NONE',  ( 0.000000000000000000, 0.000000000000000000, 1.000000000000000000 ) ) ;
#29965=CARTESIAN_POINT ( 'NONE',  ( 21.09785597605720753, -5.098646251524523443, 47.04930799450052348 ) ) ;
#29967=DIRECTION ( 'NONE',  ( -1.224646799147353207E-16, 0.000000000000000000, -1.000000000000000000 ) ) ;
#30030=CYLINDRICAL_SURFACE ( 'NONE', #20916, 31.00000000000000000 ) ;
#30033=CARTESIAN_POINT ( 'NONE',  ( -16.40214402394279958, -5.098646251524523443, 47.04930799450052348 ) ) ;
#30057=FACE_OUTER_BOUND ( 'NONE', #22491, .T. ) ;
#30066=DIRECTION ( 'NONE',  ( -0.000000000000000000, -1.000000000000000000, 0.000000000000000000 ) ) ;
#30076=DIRECTION ( 'NONE',  ( -0.000000000000000000, -1.000000000000000000, 0.000000000000000000 ) ) ;
#30077=CARTESIAN_POINT ( 'NONE',  ( 21.09785597605720753, -5.098646251524523443, 47.04930799450052348 ) ) ;
#30080=AXIS2_PLACEMENT_3D ( 'NONE', #15834, #1051, #31256 ) ;
#30095=DIRECTION ( 'NONE',  ( -1.000000000000000000, 0.000000000000000000, 0.000000000000000000 ) ) ;
#30100=ORIENTED_EDGE ( 'NONE', *, *, #17420, .T. ) ;
#30105=DIRECTION ( 'NONE',  ( -1.000000000000000000, 0.000000000000000000, 0.000000000000000000 ) ) ;
#30106=CARTESIAN_POINT ( 'NONE',  ( -12.40214402394279603, 13.86454579224779948, 47.04930799450052348 ) ) ;
#30114=EDGE_CURVE ( 'NONE', #20299, #5196, #32385, .T. ) ;
#30126=CYLINDRICAL_SURFACE ( 'NONE', #6383, 19.50000000000000000 ) ;
#30132=ORIENTED_EDGE ( 'NONE', *, *, #11524, .T. ) ;
#30136=EDGE_LOOP ( 'NONE', ( #26224, #26916, #3085, #15363 ) ) ;
#30147=AXIS2_PLACEMENT_3D ( 'NONE', #27186, #16680, #19634 ) ;
#30149=AXIS2_PLACEMENT_3D ( 'NONE', #8186, #20649, #18175 ) ;
#30163=DIRECTION ( 'NONE',  ( -0.000000000000000000, -1.000000000000000000, 0.000000000000000000 ) ) ;
#30215=AXIS2_PLACEMENT_3D ( 'NONE', #6737, #11993, #6906 ) ;
#30219=ADVANCED_FACE ( 'NONE', ( #12534 ), #9578, .F. ) ;
#30221=EDGE_CURVE ( 'NONE', #4851, #21342, #2199, .T. ) ;
#30243=ORIENTED_EDGE ( 'NONE', *, *, #31910, .T. ) ;
#30244=ADVANCED_FACE ( 'NONE', ( #29760 ), #13223, .F. ) ;
#30245=FACE_OUTER_BOUND ( 'NONE', #4861, .T. ) ;
#30263=DIRECTION ( 'NONE',  ( -1.000000000000000000, 0.000000000000000000, 0.000000000000000000 ) ) ;
#30276=FACE_OUTER_BOUND ( 'NONE', #18247, .T. ) ;
#30287=DIRECTION ( 'NONE',  ( -0.000000000000000000, -1.000000000000000000, 0.000000000000000000 ) ) ;
#30290=ORIENTED_EDGE ( 'NONE', *, *, #31390, .T. ) ;
#30296=DIRECTION ( 'NONE',  ( -1.000000000000000000, 0.000000000000000000, 0.000000000000000000 ) ) ;
#30303=VECTOR ( 'NONE', #1935, 1000.000000000000114 ) ;
#30308=ORIENTED_EDGE ( 'NONE', *, *, #20470, .F. ) ;
#30314=CARTESIAN_POINT ( 'NONE',  ( 40.09785597605721108, 14.86454579224779948, 47.04930799450052348 ) ) ;
#30323=DIRECTION ( 'NONE',  ( -0.000000000000000000, -1.000000000000000000, 0.000000000000000000 ) ) ;
#30332=CIRCLE ( 'NONE', #17200, 2.000000000000001776 ) ;
#30337=ORIENTED_EDGE ( 'NONE', *, *, #21785, .T. ) ;
#30344=EDGE_CURVE ( 'NONE', #5510, #6508, #5392, .T. ) ;
#30354=ORIENTED_EDGE ( 'NONE', *, *, #2605, .F. ) ;
#30360=DIRECTION ( 'NONE',  ( -1.000000000000000000, 0.000000000000000000, 0.000000000000000000 ) ) ;
#30379=EDGE_LOOP ( 'NONE', ( #11639, #28814, #1618, #22411 ) ) ;
#30397=DIRECTION ( 'NONE',  ( -0.000000000000000000, -1.000000000000000000, 0.000000000000000000 ) ) ;
#30407=DIRECTION ( 'NONE',  ( -1.000000000000000000, 0.000000000000000000, 0.000000000000000000 ) ) ;
#30410=VECTOR ( 'NONE', #14841, 999.9999999999998863 ) ;
#30414=AXIS2_PLACEMENT_3D ( 'NONE', #10414, #7472, #15648 ) ;
#30417=ORIENTED_EDGE ( 'NONE', *, *, #27349, .T. ) ;
#30423=DIRECTION ( 'NONE',  ( -1.000000000000000000, 0.000000000000000000, 0.000000000000000000 ) ) ;
#30428=EDGE_CURVE ( 'NONE', #19129, #27059, #32149, .T. ) ;
#30429=TOROIDAL_SURFACE ( 'NONE', #15724, 46.69263079098917046, 1.200000000000001954 ) ;
#30440=EDGE_CURVE ( 'NONE', #13364, #23946, #27052, .T. ) ;
#30452=DIRECTION ( 'NONE',  ( -1.000000000000000000, 0.000000000000000000, 0.000000000000000000 ) ) ;
#30467=CIRCLE ( 'NONE', #17866, 31.50000000000000000 ) ;
#30472=EDGE_CURVE ( 'NONE', #7619, #18982, #24231, .T. ) ;
#30512=EDGE_CURVE ( 'NONE', #7100, #15722, #26319, .T. ) ;
#30548=CIRCLE ( 'NONE', #9051, 0.4000000000000010214 ) ;
#30554=DIRECTION ( 'NONE',  ( -1.000000000000000000, 0.000000000000000000, 0.000000000000000000 ) ) ;
#30565=CARTESIAN_POINT ( 'NONE',  ( 21.09785597605720753, 14.86454579224779948, 47.04930799450052348 ) ) ;
#30581=AXIS2_PLACEMENT_3D ( 'NONE', #2622, #22642, #12970 ) ;
#30591=CIRCLE ( 'NONE', #20105, 1.499999999999999556 ) ;
#30597=AXIS2_PLACEMENT_3D ( 'NONE', #3716, #927, #28663 ) ;
#30599=DIRECTION ( 'NONE',  ( -0.000000000000000000, -1.000000000000000000, 0.000000000000000000 ) ) ;
#30602=CARTESIAN_POINT ( 'NONE',  ( 21.09785597605720753, 14.86454579224779948, 47.04930799450052348 ) ) ;
#30603=CARTESIAN_POINT ( 'NONE',  ( 58.09785597605721108, 13.86454579224779948, 47.04930799450051637 ) ) ;
#30613=DIRECTION ( 'NONE',  ( -1.000000000000000000, 0.000000000000000000, 0.000000000000000000 ) ) ;
#30614=EDGE_LOOP ( 'NONE', ( #28157, #15612, #1052, #20106 ) ) ;
#30617=DIRECTION ( 'NONE',  ( -1.000000000000000000, 0.000000000000000000, 0.000000000000000000 ) ) ;
#30621=CARTESIAN_POINT ( 'NONE',  ( 21.09785597605720753, 17.36474115922713324, 47.04930799450052348 ) ) ;
#30629=EDGE_CURVE ( 'NONE', #20299, #19168, #24758, .T. ) ;
#30678=ADVANCED_FACE ( 'NONE', ( #3880 ), #20577, .F. ) ;
#30684=CARTESIAN_POINT ( 'NONE',  ( 21.09785597605720753, 14.86454579224779948, 47.04930799450052348 ) ) ;
#30690=CARTESIAN_POINT ( 'NONE',  ( 21.09785597605720753, 15.57592086119046826, 47.04930799450052348 ) ) ;
#30694=ORIENTED_EDGE ( 'NONE', *, *, #29128, .T. ) ;
#30695=DIRECTION ( 'NONE',  ( -0.000000000000000000, -1.000000000000000000, 0.000000000000000000 ) ) ;
#30721=EDGE_CURVE ( 'NONE', #4851, #10602, #10646, .T. ) ;
#30726=DIRECTION ( 'NONE',  ( -0.000000000000000000, -1.000000000000000000, 0.000000000000000000 ) ) ;
#30727=CARTESIAN_POINT ( 'NONE',  ( 36.33160203359362583, 14.46497581658974063, 47.04930799450052348 ) ) ;
#30732=CARTESIAN_POINT ( 'NONE',  ( 21.09785597605720753, -5.098646251524523443, 47.04930799450052348 ) ) ;
#30743=LINE ( 'NONE', #7767, #17296 ) ;
#30750=CIRCLE ( 'NONE', #2443, 1.499999999999997780 ) ;
#30758=ORIENTED_EDGE ( 'NONE', *, *, #27349, .F. ) ;
#30759=DIRECTION ( 'NONE',  ( 1.000000000000000000, 0.000000000000000000, 0.000000000000000000 ) ) ;
#30777=CARTESIAN_POINT ( 'NONE',  ( 58.59785597605721108, -5.098646251524523443, 47.04930799450051637 ) ) ;
#30783=ORIENTED_EDGE ( 'NONE', *, *, #25664, .T. ) ;
#30794=AXIS2_PLACEMENT_3D ( 'NONE', #28147, #5651, #8123 ) ;
#30801=ORIENTED_EDGE ( 'NONE', *, *, #18846, .T. ) ;
#30813=CARTESIAN_POINT ( 'NONE',  ( 1.597855976057205973, -5.098646251524523443, 47.04930799450052348 ) ) ;
#30817=DIRECTION ( 'NONE',  ( -1.000000000000000000, 0.000000000000000000, 0.000000000000000000 ) ) ;
#30819=ORIENTED_EDGE ( 'NONE', *, *, #30221, .F. ) ;
#30826=CIRCLE ( 'NONE', #4077, 25.50000000000000355 ) ;
#30829=ORIENTED_EDGE ( 'NONE', *, *, #9543, .T. ) ;
#30844=DIRECTION ( 'NONE',  ( -1.000000000000000000, 0.000000000000000000, 0.000000000000000000 ) ) ;
#30847=VECTOR ( 'NONE', #27009, 1000.000000000000000 ) ;
#30848=DIRECTION ( 'NONE',  ( -1.000000000000000000, 0.000000000000000000, 0.000000000000000000 ) ) ;
#30851=VERTEX_POINT ( 'NONE', #21420 ) ;
#30855=CARTESIAN_POINT ( 'NONE',  ( 38.59785597605721108, 14.86454579224779948, 47.04930799450052348 ) ) ;
#30869=CARTESIAN_POINT ( 'NONE',  ( 21.09785597605720753, -5.098646251524523443, 47.04930799450052348 ) ) ;
#30881=CARTESIAN_POINT ( 'NONE',  ( 36.38461588890405096, 14.98269195386757602, 47.04930799450052348 ) ) ;
#30882=DIRECTION ( 'NONE',  ( -1.000000000000000000, 0.000000000000000000, 0.000000000000000000 ) ) ;
#30896=VERTEX_POINT ( 'NONE', #14544 ) ;
#30904=ORIENTED_EDGE ( 'NONE', *, *, #10015, .T. ) ;
#30932=DIRECTION ( 'NONE',  ( -0.000000000000000000, -1.000000000000000000, 0.000000000000000000 ) ) ;
#30946=AXIS2_PLACEMENT_3D ( 'NONE', #11301, #1768, #26552 ) ;
#30951=CIRCLE ( 'NONE', #547, 1.499999999999997780 ) ;
#31008=FACE_OUTER_BOUND ( 'NONE', #17997, .T. ) ;
#31019=AXIS2_PLACEMENT_3D ( 'NONE', #26522, #6662, #2057 ) ;
#31035=ORIENTED_EDGE ( 'NONE', *, *, #22205, .F. ) ;
#31039=CARTESIAN_POINT ( 'NONE',  ( 21.09785597605720753, 14.86454579224779948, 47.04930799450052348 ) ) ;
#31040=DIRECTION ( 'NONE',  ( -0.000000000000000000, -1.000000000000000000, 0.000000000000000000 ) ) ;
#31044=DIRECTION ( 'NONE',  ( -0.000000000000000000, -1.000000000000000000, 0.000000000000000000 ) ) ;
#31048=ORIENTED_EDGE ( 'NONE', *, *, #30721, .T. ) ;
#31053=DIRECTION ( 'NONE',  ( -0.000000000000000000, -1.000000000000000000, 0.000000000000000000 ) ) ;
#31082=VECTOR ( 'NONE', #8174, 1000.000000000000000 ) ;
#31086=ORIENTED_EDGE ( 'NONE', *, *, #15041, .T. ) ;
#31096=CARTESIAN_POINT ( 'NONE',  ( -0.4021440239427923058, -5.098646251524523443, 47.04930799450052348 ) ) ;
#31105=CIRCLE ( 'NONE', #16393, 0.9999999999999940048 ) ;
#31118=CYLINDRICAL_SURFACE ( 'NONE', #10901, 13.00178401536290806 ) ;
#31124=DIRECTION ( 'NONE',  ( -0.000000000000000000, -1.000000000000000000, 0.000000000000000000 ) ) ;
#31136=CIRCLE ( 'NONE', #11727, 0.2000000000000005107 ) ;
#31141=ORIENTED_EDGE ( 'NONE', *, *, #29126, .T. ) ;
#31203=ORIENTED_EDGE ( 'NONE', *, *, #20964, .T. ) ;
#31204=CARTESIAN_POINT ( 'NONE',  ( -33.00214402394279745, 14.36454579224779948, 47.04930799450052348 ) ) ;
#31223=AXIS2_PLACEMENT_3D ( 'NONE', #19315, #3904, #29340 ) ;
#31234=ORIENTED_EDGE ( 'NONE', *, *, #26593, .T. ) ;
#31243=DIRECTION ( 'NONE',  ( -0.000000000000000000, -1.000000000000000000, 0.000000000000000000 ) ) ;
#31252=FACE_OUTER_BOUND ( 'NONE', #23737, .T. ) ;
#31256=DIRECTION ( 'NONE',  ( -1.000000000000000000, 0.000000000000000000, 0.000000000000000000 ) ) ;
#31267=EDGE_CURVE ( 'NONE', #13235, #12313, #16933, .T. ) ;
#31272=DIRECTION ( 'NONE',  ( -0.000000000000000000, -1.000000000000000000, 0.000000000000000000 ) ) ;
#31273=EDGE_CURVE ( 'NONE', #30896, #163, #8923, .T. ) ;
#31290=CARTESIAN_POINT ( 'NONE',  ( 21.09785597605720753, 13.86454579224779948, 47.04930799450052348 ) ) ;
#31296=ADVANCED_FACE ( 'NONE', ( #26490 ), #10144, .F. ) ;
#31299=AXIS2_PLACEMENT_3D ( 'NONE', #20523, #22824, #30554 ) ;
#31306=ADVANCED_FACE ( 'NONE', ( #2684 ), #29535, .T. ) ;
#31310=ORIENTED_EDGE ( 'NONE', *, *, #7457, .T. ) ;
#31318=ORIENTED_EDGE ( 'NONE', *, *, #27698, .F. ) ;
#31319=ORIENTED_EDGE ( 'NONE', *, *, #17407, .F. ) ;
#31321=VERTEX_POINT ( 'NONE', #25167 ) ;
#31325=FACE_OUTER_BOUND ( 'NONE', #23740, .T. ) ;
#31327=FACE_OUTER_BOUND ( 'NONE', #620, .T. ) ;
#31341=CARTESIAN_POINT ( 'NONE',  ( 62.59785597605721819, 14.86454579224779948, 47.04930799450051637 ) ) ;
#31342=AXIS2_PLACEMENT_3D ( 'NONE', #16804, #1875, #11890 ) ;
#31345=EDGE_CURVE ( 'NONE', #26091, #294, #19010, .T. ) ;
#31348=AXIS2_PLACEMENT_3D ( 'NONE', #3432, #21142, #10515 ) ;
#31354=AXIS2_PLACEMENT_3D ( 'NONE', #15825, #10424, #23043 ) ;
#31361=ORIENTED_EDGE ( 'NONE', *, *, #19783, .T. ) ;
#31366=ORIENTED_EDGE ( 'NONE', *, *, #4038, .F. ) ;
#31383=ORIENTED_EDGE ( 'NONE', *, *, #17705, .F. ) ;
#31390=EDGE_CURVE ( 'NONE', #22149, #27481, #9622, .T. ) ;
#31397=AXIS2_PLACEMENT_3D ( 'NONE', #3080, #634, #8341 ) ;
#31398=AXIS2_PLACEMENT_3D ( 'NONE', #6144, #29118, #21226 ) ;
#31401=DIRECTION ( 'NONE',  ( -1.000000000000000000, 0.000000000000000000, 0.000000000000000000 ) ) ;
#31403=CARTESIAN_POINT ( 'NONE',  ( 21.09785597605720753, -5.098646251524523443, 47.04930799450052348 ) ) ;
#31410=LINE ( 'NONE', #21863, #19426 ) ;
#31450=CARTESIAN_POINT ( 'NONE',  ( 21.09785597605720753, 13.86454579224779948, 47.04930799450052348 ) ) ;
#31451=DIRECTION ( 'NONE',  ( -1.000000000000000000, 0.000000000000000000, 0.000000000000000000 ) ) ;
#31454=DIRECTION ( 'NONE',  ( -1.000000000000000000, 0.000000000000000000, 0.000000000000000000 ) ) ;
#31475=CIRCLE ( 'NONE', #20465, 31.50000000000000000 ) ;
#31495=CARTESIAN_POINT ( 'NONE',  ( 21.09785597605720753, 13.86454579224779948, 47.04930799450052348 ) ) ;
#31496=CIRCLE ( 'NONE', #26775, 0.1999999999999987899 ) ;
#31507=EDGE_CURVE ( 'NONE', #25220, #663, #21151, .T. ) ;
#31529=AXIS2_PLACEMENT_3D ( 'NONE', #29801, #30287, #17639 ) ;
#31568=ORIENTED_EDGE ( 'NONE', *, *, #19784, .T. ) ;
#31576=AXIS2_PLACEMENT_3D ( 'NONE', #10152, #12943, #29850 ) ;
#31605=CARTESIAN_POINT ( 'NONE',  ( 64.59785597605720397, -5.098646251524523443, 47.04930799450051637 ) ) ;
#31617=ORIENTED_EDGE ( 'NONE', *, *, #10614, .F. ) ;
#31629=EDGE_LOOP ( 'NONE', ( #5019, #15533, #30337, #10894 ) ) ;
#31648=EDGE_CURVE ( 'NONE', #5653, #3892, #198, .T. ) ;
#31653=CYLINDRICAL_SURFACE ( 'NONE', #22817, 13.00178401536290806 ) ;
#31666=ORIENTED_EDGE ( 'NONE', *, *, #29805, .T. ) ;
#31668=EDGE_CURVE ( 'NONE', #6508, #5510, #14357, .T. ) ;
#31674=DIRECTION ( 'NONE',  ( -0.000000000000000000, 1.000000000000000000, 0.000000000000000000 ) ) ;
#31676=ORIENTED_EDGE ( 'NONE', *, *, #22568, .F. ) ;
#31677=TOROIDAL_SURFACE ( 'NONE', #234, 54.10000000000000142, 0.1999999999999993727 ) ;
#31701=DIRECTION ( 'NONE',  ( 1.000000000000000000, 0.000000000000000000, 0.000000000000000000 ) ) ;
#31745=VERTEX_POINT ( 'NONE', #24634 ) ;
#31756=ADVANCED_FACE ( 'NONE', ( #22167 ), #14957, .T. ) ;
#31760=VERTEX_POINT ( 'NONE', #17725 ) ;
#31768=DIRECTION ( 'NONE',  ( -1.000000000000000000, 0.000000000000000000, 0.000000000000000000 ) ) ;
#31772=EDGE_LOOP ( 'NONE', ( #996, #1256, #19146, #12069 ) ) ;
#31783=CARTESIAN_POINT ( 'NONE',  ( 64.09785597605720397, -5.098646251524523443, 47.04930799450051637 ) ) ;
#31836=EDGE_CURVE ( 'NONE', #15810, #30896, #13374, .T. ) ;
#31838=TOROIDAL_SURFACE ( 'NONE', #26069, 20.49999999999999645, 0.9999999999999974465 ) ;
#31840=( NAMED_UNIT ( * ) PLANE_ANGLE_UNIT ( ) SI_UNIT ( $, .RADIAN. ) );
#31872=VERTEX_POINT ( 'NONE', #5431 ) ;
#31875=EDGE_CURVE ( 'NONE', #31760, #1013, #22815, .T. ) ;
#31890=ORIENTED_EDGE ( 'NONE', *, *, #4944, .T. ) ;
#31896=EDGE_LOOP ( 'NONE', ( #22241, #23876, #27518, #6027 ) ) ;
#31901=ADVANCED_FACE ( 'NONE', ( #25385 ), #3399, .F. ) ;
#31910=EDGE_CURVE ( 'NONE', #23289, #21342, #6037, .T. ) ;
#31921=VERTEX_POINT ( 'NONE', #275 ) ;
#31929=DIRECTION ( 'NONE',  ( -1.000000000000000000, 0.000000000000000000, 0.000000000000000000 ) ) ;
#31933=DIRECTION ( 'NONE',  ( 1.000000000000000000, 0.000000000000000000, 0.000000000000000000 ) ) ;
#31934=DIRECTION ( 'NONE',  ( -1.000000000000000000, 0.000000000000000000, 0.000000000000000000 ) ) ;
#31948=TOROIDAL_SURFACE ( 'NONE', #14666, 13.20178401536290913, 0.2000000000000002609 ) ;
#31983=CARTESIAN_POINT ( 'NONE',  ( 21.09785597605720753, 17.16467605102632632, 47.04930799450052348 ) ) ;
#31988=CIRCLE ( 'NONE', #30946, 33.50000000000000000 ) ;
#31998=CARTESIAN_POINT ( 'NONE',  ( 44.59785597605720397, 14.86454579224779948, 47.04930799450052348 ) ) ;
#32011=ORIENTED_EDGE ( 'NONE', *, *, #20470, .T. ) ;
#32019=AXIS2_PLACEMENT_3D ( 'NONE', #21263, #772, #21102 ) ;
#32032=EDGE_LOOP ( 'NONE', ( #238, #27939, #31086, #4976 ) ) ;
#32051=( NAMED_UNIT ( * ) PLANE_ANGLE_UNIT ( ) SI_UNIT ( $, .RADIAN. ) );
#32062=DIRECTION ( 'NONE',  ( -0.000000000000000000, -1.000000000000000000, 0.000000000000000000 ) ) ;
#32073=CIRCLE ( 'NONE', #12135, 0.5000000000000004441 ) ;
#32095=LINE ( 'NONE', #4677, #26936 ) ;
#32098=DIRECTION ( 'NONE',  ( -1.000000000000000000, 0.000000000000000000, 0.000000000000000000 ) ) ;
#32102=CARTESIAN_POINT ( 'NONE',  ( 36.45249510457200870, 15.11603238453479037, 47.04930799450052348 ) ) ;
#32130=ORIENTED_EDGE ( 'NONE', *, *, #8252, .T. ) ;
#32149=LINE ( 'NONE', #4246, #646 ) ;
#32158=AXIS2_PLACEMENT_3D ( 'NONE', #22208, #12212, #32394 ) ;
#32177=AXIS2_PLACEMENT_3D ( 'NONE', #706, #21038, #8105 ) ;
#32192=CARTESIAN_POINT ( 'NONE',  ( 75.39785597605720113, -5.098646251524523443, 47.04930799450051637 ) ) ;
#32198=DIRECTION ( 'NONE',  ( -0.000000000000000000, -1.000000000000000000, 0.000000000000000000 ) ) ;
#32226=TOROIDAL_SURFACE ( 'NONE', #29071, 29.50000000000000355, 2.000000000000001776 ) ;
#32229=DIRECTION ( 'NONE',  ( 0.000000000000000000, 0.000000000000000000, 1.000000000000000000 ) ) ;
#32234=TOROIDAL_SURFACE ( 'NONE', #2357, 46.75000000000000000, 1.290569415042097656 ) ;
#32277=AXIS2_PLACEMENT_3D ( 'NONE', #9891, #20371, #27287 ) ;
#32281=EDGE_CURVE ( 'NONE', #25889, #23946, #28057, .T. ) ;
#32305=DIRECTION ( 'NONE',  ( -0.000000000000000000, -1.000000000000000000, 0.000000000000000000 ) ) ;
#32311=TOROIDAL_SURFACE ( 'NONE', #18668, 46.75000000000000000, 1.290569415042097656 ) ;
#32316=ORIENTED_EDGE ( 'NONE', *, *, #1709, .T. ) ;
#32321=CIRCLE ( 'NONE', #345, 13.20165371409683885 ) ;
#32338=CARTESIAN_POINT ( 'NONE',  ( -15.90214402394279958, 14.86454579224779948, 47.04930799450052348 ) ) ;
#32377=ORIENTED_EDGE ( 'NONE', *, *, #25819, .F. ) ;
#32385=LINE ( 'NONE', #7763, #17937 ) ;
#32391=CIRCLE ( 'NONE', #31348, 13.20165371409683885 ) ;
#32394=DIRECTION ( 'NONE',  ( -1.000000000000000000, 0.000000000000000000, 0.000000000000000000 ) ) ;
#32410=AXIS2_PLACEMENT_3D ( 'NONE', #11098, #28488, #25535 ) ;
#32414=TOROIDAL_SURFACE ( 'NONE', #31354, 54.10000000000000142, 0.1999999999999994282 ) ;
#32435=PRODUCT_DEFINITION_CONTEXT ( 'detailed design', #9095, 'design' ) ;
#32436=AXIS2_PLACEMENT_3D ( 'NONE', #21239, #31272, #6317 ) ;
#32441=EDGE_CURVE ( 'NONE', #490, #24509, #24407, .T. ) ;
#32446=DIRECTION ( 'NONE',  ( -0.000000000000000000, -1.000000000000000000, 0.000000000000000000 ) ) ;
#32469=FACE_OUTER_BOUND ( 'NONE', #14809, .T. ) ;
#32474=AXIS2_PLACEMENT_3D ( 'NONE', #17719, #20508, #28069 ) ;
#32523=COLOUR_RGB('Sky Blue',0.24,0.69,0.87);
#32524=FILL_AREA_STYLE_COLOUR('',#32523);
#32525=FILL_AREA_STYLE('',(#32524));
#32526=SURFACE_STYLE_FILL_AREA(#32525);
#32527=SURFACE_SIDE_STYLE('',(#32526));
#32528=SURFACE_STYLE_USAGE(.BOTH.,#32527);
#32529=PRESENTATION_STYLE_ASSIGNMENT((#32528));
ENDSEC;
END-ISO-10303-21;
